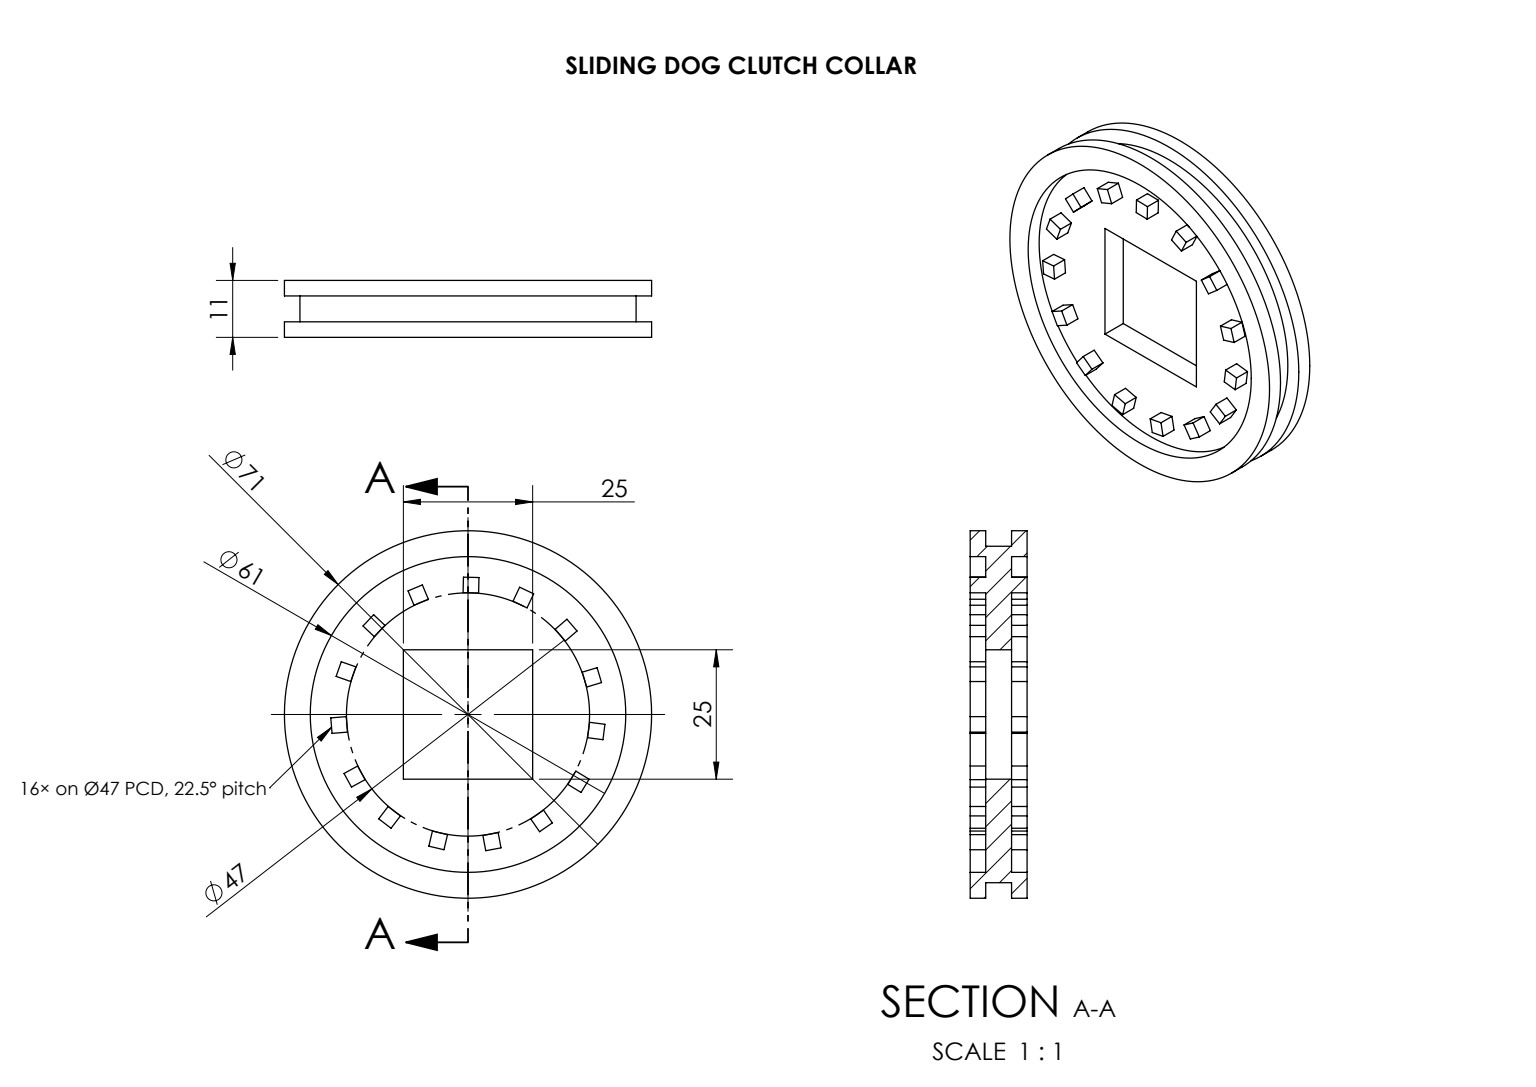
ISO-10303-21;
HEADER;
FILE_DESCRIPTION (('STEP AP214'),
    '1' );
FILE_NAME ('Sliding Dog Clutch Collar.step',
    '2026-10-08T09:53:37',
    ( '' ),
    ( '' ),
    'SwSTEP 2.0',
    'SolidWorks 2026',
    '' );
FILE_SCHEMA (( 'AUTOMOTIVE_DESIGN' ));
ENDSEC;

DATA;
#12=CARTESIAN_POINT ( 'NONE',  ( 20.85212586905262100, -130.9402397935870965, 2.500000000000000000 ) ) ;
#51=EDGE_CURVE ( 'NONE', #68933, #53084, #10085, .T. ) ;
#57=DIRECTION ( 'NONE',  ( -0.9966891607226785466, -0.08130631524009969413, 0.000000000000000000 ) ) ;
#59=DIRECTION ( 'NONE',  ( -0.3311129884571295534, -0.9435911131814398445, 0.000000000000000000 ) ) ;
#64=CARTESIAN_POINT ( 'NONE',  ( -26.29030328629083968, -123.6496510949466341, -5.500000000000000000 ) ) ;
#71=FACE_OUTER_BOUND ( 'NONE', #8361, .T. ) ;
#105=VERTEX_POINT ( 'NONE', #27751 ) ;
#152=CARTESIAN_POINT ( 'NONE',  ( -18.24502636017238899, -100.7225776329765665, 5.500000000000000000 ) ) ;
#170=ORIENTED_EDGE ( 'NONE', *, *, #48054, .T. ) ;
#195=DIRECTION ( 'NONE',  ( -0.000000000000000000, -0.000000000000000000, 1.000000000000000000 ) ) ;
#208=CARTESIAN_POINT ( 'NONE',  ( -0.7800914985199643992, -121.2811936832255100, 2.500000000000000000 ) ) ;
#210=CARTESIAN_POINT ( 'NONE',  ( 11.41210121379328335, -99.40233154247455616, 5.500000000000000000 ) ) ;
#218=EDGE_LOOP ( 'NONE', ( #22969, #71308, #32265, #23683 ) ) ;
#224=ADVANCED_FACE ( 'NONE', ( #20004 ), #64049, .F. ) ;
#245=VECTOR ( 'NONE', #9252, 1000.000000000000000 ) ;
#248=CARTESIAN_POINT ( 'NONE',  ( -16.06301359042743115, -102.7814171781257357, 2.500000000000000000 ) ) ;
#265=PLANE ( 'NONE',  #60728 ) ;
#266=CARTESIAN_POINT ( 'NONE',  ( -8.826826895187510402, -94.96827758698185562, 5.500000000000000000 ) ) ;
#268=ORIENTED_EDGE ( 'NONE', *, *, #56458, .T. ) ;
#303=EDGE_CURVE ( 'NONE', #64095, #48732, #3130, .T. ) ;
#384=CARTESIAN_POINT ( 'NONE',  ( 3.429551818649054340, -146.3199197248623875, 5.500000000000000000 ) ) ;
#386=LINE ( 'NONE', #68776, #73091 ) ;
#390=LINE ( 'NONE', #68413, #20038 ) ;
#395=CARTESIAN_POINT ( 'NONE',  ( 22.63442173698368620, -133.7816164738524378, -2.500000000000000000 ) ) ;
#401=ORIENTED_EDGE ( 'NONE', *, *, #30678, .T. ) ;
#481=FACE_OUTER_BOUND ( 'NONE', #34293, .T. ) ;
#549=DIRECTION ( 'NONE',  ( -0.3853207896976547642, 0.9227826878668540234, 0.000000000000000000 ) ) ;
#565=EDGE_CURVE ( 'NONE', #23559, #52552, #27876, .T. ) ;
#567=VECTOR ( 'NONE', #11381, 1000.000000000000000 ) ;
#580=FACE_OUTER_BOUND ( 'NONE', #12043, .T. ) ;
#591=CIRCLE ( 'NONE', #53356, 35.50000000000000711 ) ;
#648=FACE_OUTER_BOUND ( 'NONE', #4489, .T. ) ;
#656=EDGE_CURVE ( 'NONE', #45592, #59758, #43789, .T. ) ;
#726=CARTESIAN_POINT ( 'NONE',  ( 9.984461079971730157, -95.40710393340120277, 5.500000000000000000 ) ) ;
#739=CARTESIAN_POINT ( 'NONE',  ( -23.54415474984308787, -120.4156646670583086, 5.500000000000000000 ) ) ;
#753=CARTESIAN_POINT ( 'NONE',  ( 26.47460221209471598, -121.8961639463267090, 5.500000000000000000 ) ) ;
#776=EDGE_LOOP ( 'NONE', ( #60937, #39384, #65729, #18843 ) ) ;
#780=LINE ( 'NONE', #58251, #57390 ) ;
#809=CARTESIAN_POINT ( 'NONE',  ( -0.8815729230226008184, -93.47222532549339746, -5.500000000000000000 ) ) ;
#811=LINE ( 'NONE', #46635, #58781 ) ;
#837=PLANE ( 'NONE',  #5857 ) ;
#854=( NAMED_UNIT ( * ) SI_UNIT ( $, .STERADIAN. ) SOLID_ANGLE_UNIT ( ) );
#860=DIRECTION ( 'NONE',  ( -0.000000000000000000, -0.000000000000000000, -1.000000000000000000 ) ) ;
#883=EDGE_CURVE ( 'NONE', #14710, #67113, #37603, .T. ) ;
#885=ORIENTED_EDGE ( 'NONE', *, *, #19699, .F. ) ;
#897=VECTOR ( 'NONE', #23392, 1000.000000000000000 ) ;
#904=DIRECTION ( 'NONE',  ( -1.000000000000000000, 0.000000000000000000, 0.000000000000000000 ) ) ;
#920=FACE_OUTER_BOUND ( 'NONE', #19157, .T. ) ;
#923=LINE ( 'NONE', #34721, #21582 ) ;
#930=VECTOR ( 'NONE', #45166, 1000.000000000000000 ) ;
#947=AXIS2_PLACEMENT_3D ( 'NONE', #33555, #73025, #5390 ) ;
#949=PLANE ( 'NONE',  #67943 ) ;
#957=ORIENTED_EDGE ( 'NONE', *, *, #41163, .T. ) ;
#967=AXIS2_PLACEMENT_3D ( 'NONE', #58203, #18343, #42767 ) ;
#973=VERTEX_POINT ( 'NONE', #6001 ) ;
#982=CARTESIAN_POINT ( 'NONE',  ( -24.50849501662245800, -109.8101191361138831, -2.500000000000000444 ) ) ;
#1018=DIRECTION ( 'NONE',  ( -0.000000000000000000, -0.000000000000000000, 1.000000000000000000 ) ) ;
#1038=VERTEX_POINT ( 'NONE', #45100 ) ;
#1040=ORIENTED_EDGE ( 'NONE', *, *, #39297, .F. ) ;
#1043=DIRECTION ( 'NONE',  ( -0.000000000000000000, -0.000000000000000000, 1.000000000000000000 ) ) ;
#1059=ORIENTED_EDGE ( 'NONE', *, *, #39337, .F. ) ;
#1087=CARTESIAN_POINT ( 'NONE',  ( 22.08297821871651934, -111.8242998470044540, 5.500000000000000000 ) ) ;
#1092=LINE ( 'NONE', #24349, #38349 ) ;
#1109=DIRECTION ( 'NONE',  ( -0.000000000000000000, -0.000000000000000000, -1.000000000000000000 ) ) ;
#1160=FACE_OUTER_BOUND ( 'NONE', #45975, .T. ) ;
#1173=VERTEX_POINT ( 'NONE', #12346 ) ;
#1184=EDGE_LOOP ( 'NONE', ( #11101, #10539, #73075, #4642 ) ) ;
#1199=VECTOR ( 'NONE', #23641, 1000.000000000000000 ) ;
#1219=CARTESIAN_POINT ( 'NONE',  ( 13.83832728059186046, -142.6495187161941089, 5.500000000000000000 ) ) ;
#1231=ORIENTED_EDGE ( 'NONE', *, *, #64365, .F. ) ;
#1253=EDGE_CURVE ( 'NONE', #62521, #29721, #66451, .T. ) ;
#1266=EDGE_CURVE ( 'NONE', #63423, #62521, #21300, .T. ) ;
#1275=CARTESIAN_POINT ( 'NONE',  ( -16.07206065793331007, -141.0698568150738197, -2.500000000000000000 ) ) ;
#1279=ORIENTED_EDGE ( 'NONE', *, *, #2361, .T. ) ;
#1296=DIRECTION ( 'NONE',  ( -0.4279312458753000703, -0.9038112904824842087, 0.000000000000000000 ) ) ;
#1340=LINE ( 'NONE', #12563, #61150 ) ;
#1343=EDGE_LOOP ( 'NONE', ( #50298, #67195, #1354, #42780 ) ) ;
#1349=ORIENTED_EDGE ( 'NONE', *, *, #68241, .T. ) ;
#1354=ORIENTED_EDGE ( 'NONE', *, *, #44246, .T. ) ;
#1372=CARTESIAN_POINT ( 'NONE',  ( -7.572224309238338336, -145.4393675041377492, -2.500000000000000444 ) ) ;
#1380=VECTOR ( 'NONE', #34980, 1000.000000000000000 ) ;
#1381=ORIENTED_EDGE ( 'NONE', *, *, #5276, .T. ) ;
#1394=ADVANCED_FACE ( 'NONE', ( #38992 ), #12165, .F. ) ;
#1438=ORIENTED_EDGE ( 'NONE', *, *, #18270, .F. ) ;
#1485=LINE ( 'NONE', #36753, #73620 ) ;
#1487=LINE ( 'NONE', #13080, #23907 ) ;
#1521=AXIS2_PLACEMENT_3D ( 'NONE', #26148, #53617, #71638 ) ;
#1537=ORIENTED_EDGE ( 'NONE', *, *, #72023, .T. ) ;
#1539=EDGE_LOOP ( 'NONE', ( #2290, #72966 ) ) ;
#1553=CARTESIAN_POINT ( 'NONE',  ( -26.53422223201112828, -120.6595836127786043, 5.500000000000000000 ) ) ;
#1598=SURFACE_STYLE_USAGE ( .BOTH. , #12090 ) ;
#1599=ORIENTED_EDGE ( 'NONE', *, *, #38387, .F. ) ;
#1602=ORIENTED_EDGE ( 'NONE', *, *, #6612, .T. ) ;
#1625=ORIENTED_EDGE ( 'NONE', *, *, #25023, .F. ) ;
#1653=ORIENTED_EDGE ( 'NONE', *, *, #66798, .T. ) ;
#1676=AXIS2_PLACEMENT_3D ( 'NONE', #49631, #3078, #56026 ) ;
#1704=VERTEX_POINT ( 'NONE', #49333 ) ;
#1707=CARTESIAN_POINT ( 'NONE',  ( 0.4301293587033142574, -121.4370068666438556, -2.500000000000000000 ) ) ;
#1722=CARTESIAN_POINT ( 'NONE',  ( -22.53294031248081808, -134.0273518838794757, -2.500000000000000000 ) ) ;
#1723=ORIENTED_EDGE ( 'NONE', *, *, #48136, .T. ) ;
#1748=CARTESIAN_POINT ( 'NONE',  ( 10.05638427806949586, -98.76043467366159234, 2.500000000000000000 ) ) ;
#1754=CARTESIAN_POINT ( 'NONE',  ( 4.903647372192503795, -146.0423547792665886, -2.500000000000000000 ) ) ;
#1765=AXIS2_PLACEMENT_3D ( 'NONE', #44988, #68289, #73165 ) ;
#1781=VERTEX_POINT ( 'NONE', #33901 ) ;
#1784=VECTOR ( 'NONE', #5629, 1000.000000000000000 ) ;
#1785=CARTESIAN_POINT ( 'NONE',  ( 30.50000000000000000, -120.0000000000000000, 2.500000000000000000 ) ) ;
#1811=ORIENTED_EDGE ( 'NONE', *, *, #51766, .F. ) ;
#1826=ORIENTED_EDGE ( 'NONE', *, *, #3341, .T. ) ;
#1835=CARTESIAN_POINT ( 'NONE',  ( -26.53422223201112828, -120.6595836127786043, 5.500000000000000000 ) ) ;
#1837=ORIENTED_EDGE ( 'NONE', *, *, #48323, .F. ) ;
#1839=DIRECTION ( 'NONE',  ( -0.7585478161175706058, -0.6516173805718078471, 0.000000000000000000 ) ) ;
#1842=FACE_OUTER_BOUND ( 'NONE', #73904, .T. ) ;
#1847=DIRECTION ( 'NONE',  ( 0.5200609990132993854, 0.8541291221503275466, -0.000000000000000000 ) ) ;
#1885=EDGE_LOOP ( 'NONE', ( #9049, #54453, #6920, #47224 ) ) ;
#1908=FACE_BOUND ( 'NONE', #36354, .T. ) ;
#1909=DIRECTION ( 'NONE',  ( -0.6862798483830533369, -0.7273375899149812085, 0.000000000000000000 ) ) ;
#1931=CARTESIAN_POINT ( 'NONE',  ( -0.8815729230226008184, -93.47222532549339746, 5.500000000000000000 ) ) ;
#1939=CARTESIAN_POINT ( 'NONE',  ( -18.12185313557660038, -104.9634299478706794, 5.500000000000000000 ) ) ;
#1956=CARTESIAN_POINT ( 'NONE',  ( -22.67106064244953245, -113.6342314410295842, 2.500000000000000000 ) ) ;
#1959=EDGE_LOOP ( 'NONE', ( #56725, #22128, #74154, #73797 ) ) ;
#1966=VERTEX_POINT ( 'NONE', #2696 ) ;
#1969=ORIENTED_EDGE ( 'NONE', *, *, #5881, .F. ) ;
#1977=ADVANCED_FACE ( 'NONE', ( #41753 ), #7186, .T. ) ;
#2011=EDGE_CURVE ( 'NONE', #44097, #4558, #30834, .T. ) ;
#2015=DIRECTION ( 'NONE',  ( -0.7585478161175716050, -0.6516173805718067369, 0.000000000000000000 ) ) ;
#2029=CARTESIAN_POINT ( 'NONE',  ( -23.30023580412278505, -123.4057321492263384, 5.500000000000000000 ) ) ;
#2040=FILL_AREA_STYLE_COLOUR ( '', #49372 ) ;
#2043=CARTESIAN_POINT ( 'NONE',  ( -11.59517495878806947, -96.12423995607481686, 5.500000000000000000 ) ) ;
#2082=ORIENTED_EDGE ( 'NONE', *, *, #60638, .T. ) ;
#2084=CARTESIAN_POINT ( 'NONE',  ( 0.6180191030787338669, -93.50720753887522108, -2.500000000000000000 ) ) ;
#2101=CARTESIAN_POINT ( 'NONE',  ( -24.94940289813038703, -237.3777120880567963, 5.500000000000000000 ) ) ;
#2107=EDGE_CURVE ( 'NONE', #22856, #34880, #48875, .T. ) ;
#2113=EDGE_CURVE ( 'NONE', #8769, #59758, #72169, .T. ) ;
#2145=ORIENTED_EDGE ( 'NONE', *, *, #64889, .T. ) ;
#2160=CARTESIAN_POINT ( 'NONE',  ( -26.29030328629083968, -123.6496510949466341, 2.500000000000000000 ) ) ;
#2173=CARTESIAN_POINT ( 'NONE',  ( 23.41451323550360186, -132.5004227906269989, -5.500000000000000000 ) ) ;
#2175=CARTESIAN_POINT ( 'NONE',  ( -1.384174031800281979, -120.5779811845464735, -2.500000000000000000 ) ) ;
#2189=DIRECTION ( 'NONE',  ( -0.9918136447140100120, 0.1276937514489704939, 0.000000000000000000 ) ) ;
#2197=ORIENTED_EDGE ( 'NONE', *, *, #69129, .F. ) ;
#2202=ORIENTED_EDGE ( 'NONE', *, *, #62936, .T. ) ;
#2290=ORIENTED_EDGE ( 'NONE', *, *, #74029, .F. ) ;
#2315=CARTESIAN_POINT ( 'NONE',  ( -15.44521549751111955, -137.7748507232956001, -2.500000000000000000 ) ) ;
#2321=EDGE_CURVE ( 'NONE', #28941, #7487, #57491, .T. ) ;
#2322=ADVANCED_FACE ( 'NONE', ( #73654 ), #10891, .F. ) ;
#2326=PLANE ( 'NONE',  #26246 ) ;
#2329=CARTESIAN_POINT ( 'NONE',  ( -20.30386590532155111, -102.9045904027214959, -2.500000000000000000 ) ) ;
#2332=VECTOR ( 'NONE', #7775, 1000.000000000000114 ) ;
#2351=CARTESIAN_POINT ( 'NONE',  ( -20.30386590532152979, -102.9045904027214959, 5.500000000000000000 ) ) ;
#2360=VECTOR ( 'NONE', #38026, 1000.000000000000000 ) ;
#2361=EDGE_CURVE ( 'NONE', #54121, #6591, #390, .T. ) ;
#2369=FACE_OUTER_BOUND ( 'NONE', #40880, .T. ) ;
#2372=ORIENTED_EDGE ( 'NONE', *, *, #7575, .T. ) ;
#2386=DIRECTION ( 'NONE',  ( -0.000000000000000000, -0.000000000000000000, -1.000000000000000000 ) ) ;
#2405=DIRECTION ( 'NONE',  ( -0.6862798483830533369, -0.7273375899149812085, 0.000000000000000000 ) ) ;
#2427=CARTESIAN_POINT ( 'NONE',  ( 24.94940289813197509, -237.3777120880564553, -5.500000000000000000 ) ) ;
#2428=DIRECTION ( 'NONE',  ( 0.6064928550163524168, 0.7950889364178788110, -0.000000000000000000 ) ) ;
#2467=DIRECTION ( 'NONE',  ( -0.000000000000000000, -0.000000000000000000, -1.000000000000000000 ) ) ;
#2505=EDGE_CURVE ( 'NONE', #6335, #6594, #41666, .T. ) ;
#2541=CARTESIAN_POINT ( 'NONE',  ( -0.7800914985199643992, -121.2811936832255100, -2.500000000000000000 ) ) ;
#2561=LINE ( 'NONE', #48369, #245 ) ;
#2568=DIRECTION ( 'NONE',  ( 0.3090169943749448977, 0.9510565162951543083, 0.000000000000000000 ) ) ;
#2579=LINE ( 'NONE', #1835, #53727 ) ;
#2597=CARTESIAN_POINT ( 'NONE',  ( -23.54415474984308432, -120.4156646670583086, -2.500000000000000000 ) ) ;
#2615=ADVANCED_FACE ( 'NONE', ( #26957 ), #2964, .F. ) ;
#2624=DIRECTION ( 'NONE',  ( -0.2867529058022035837, 0.9580045777625452175, 0.000000000000000000 ) ) ;
#2634=ORIENTED_EDGE ( 'NONE', *, *, #24041, .F. ) ;
#2635=CARTESIAN_POINT ( 'NONE',  ( 12.13205353604972991, -140.1820037904669789, 5.500000000000000000 ) ) ;
#2639=CARTESIAN_POINT ( 'NONE',  ( -3.961125083139900749, -143.2122702051246677, 5.500000000000000000 ) ) ;
#2641=CARTESIAN_POINT ( 'NONE',  ( 12.13205353604972991, -140.1820037904669789, 5.500000000000000000 ) ) ;
#2654=VERTEX_POINT ( 'NONE', #43173 ) ;
#2667=DIRECTION ( 'NONE',  ( -0.1850432970638682395, 0.9827303690289280746, 0.000000000000000000 ) ) ;
#2671=EDGE_CURVE ( 'NONE', #22209, #16806, #61189, .T. ) ;
#2689=CARTESIAN_POINT ( 'NONE',  ( 32.50000000000000000, -120.0000000000000000, 2.500000000000000000 ) ) ;
#2696=CARTESIAN_POINT ( 'NONE',  ( 24.95699195200416654, -110.9640411295978595, 2.500000000000000000 ) ) ;
#2712=CARTESIAN_POINT ( 'NONE',  ( -0.1219594728601508804, -118.5049662589159567, -2.500000000000000000 ) ) ;
#2717=DIRECTION ( 'NONE',  ( -0.000000000000000000, -0.000000000000000000, -1.000000000000000000 ) ) ;
#2726=EDGE_LOOP ( 'NONE', ( #54837, #44802, #69623, #30782 ) ) ;
#2730=EDGE_LOOP ( 'NONE', ( #43648, #11853, #10232, #41324 ) ) ;
#2752=FACE_OUTER_BOUND ( 'NONE', #72336, .T. ) ;
#2755=DIRECTION ( 'NONE',  ( 0.02332147558787931590, 0.9997280174009348652, -0.000000000000000000 ) ) ;
#2758=EDGE_CURVE ( 'NONE', #7483, #63916, #28822, .T. ) ;
#2759=CARTESIAN_POINT ( 'NONE',  ( 0.9774260708577211521, -121.1378217241763622, 2.500000000000000000 ) ) ;
#2762=ORIENTED_EDGE ( 'NONE', *, *, #2758, .T. ) ;
#2775=DIRECTION ( 'NONE',  ( 0.000000000000000000, 0.000000000000000000, -1.000000000000000000 ) ) ;
#2784=CARTESIAN_POINT ( 'NONE',  ( 21.07894319797337701, -103.8699611390234878, -5.500000000000000000 ) ) ;
#2800=VERTEX_POINT ( 'NONE', #21694 ) ;
#2808=ORIENTED_EDGE ( 'NONE', *, *, #40826, .F. ) ;
#2845=ORIENTED_EDGE ( 'NONE', *, *, #10162, .F. ) ;
#2868=AXIS2_PLACEMENT_3D ( 'NONE', #12120, #35427, #47091 ) ;
#2902=VERTEX_POINT ( 'NONE', #45779 ) ;
#2915=DIRECTION ( 'NONE',  ( -0.000000000000000000, -0.000000000000000000, -1.000000000000000000 ) ) ;
#2924=CARTESIAN_POINT ( 'NONE',  ( -30.50000000000000000, -120.0000000000000000, 2.500000000000000000 ) ) ;
#2944=CARTESIAN_POINT ( 'NONE',  ( -20.62008904684763166, -131.2721749321093512, 2.500000000000000000 ) ) ;
#2957=EDGE_CURVE ( 'NONE', #62465, #52552, #27369, .T. ) ;
#2964=PLANE ( 'NONE',  #49843 ) ;
#2978=DIRECTION ( 'NONE',  ( 0.9580045777625452175, 0.2867529058022035837, -0.000000000000000000 ) ) ;
#2990=DIRECTION ( 'NONE',  ( -0.7950889364178798102, 0.6064928550163511956, 0.000000000000000000 ) ) ;
#3010=ORIENTED_EDGE ( 'NONE', *, *, #53161, .F. ) ;
#3022=VERTEX_POINT ( 'NONE', #62360 ) ;
#3034=CARTESIAN_POINT ( 'NONE',  ( 26.09152095774781799, -124.8716048804687375, 5.500000000000000000 ) ) ;
#3036=LINE ( 'NONE', #9373, #47208 ) ;
#3037=CARTESIAN_POINT ( 'NONE',  ( 13.83832728059186046, -142.6495187161941089, -5.500000000000000000 ) ) ;
#3045=FACE_OUTER_BOUND ( 'NONE', #46790, .T. ) ;
#3051=ORIENTED_EDGE ( 'NONE', *, *, #65354, .T. ) ;
#3078=DIRECTION ( 'NONE',  ( 0.7585478161175706058, 0.6516173805718080692, -0.000000000000000000 ) ) ;
#3096=ORIENTED_EDGE ( 'NONE', *, *, #22042, .T. ) ;
#3099=LINE ( 'NONE', #53462, #15602 ) ;
#3103=EDGE_CURVE ( 'NONE', #27761, #71554, #57819, .T. ) ;
#3126=CARTESIAN_POINT ( 'NONE',  ( 21.07894319797337701, -103.8699611390234878, 5.500000000000000000 ) ) ;
#3130=LINE ( 'NONE', #61360, #42832 ) ;
#3142=CARTESIAN_POINT ( 'NONE',  ( 21.07894319797337701, -103.8699611390234878, 5.500000000000000000 ) ) ;
#3144=LINE ( 'NONE', #43723, #13744 ) ;
#3149=ORIENTED_EDGE ( 'NONE', *, *, #18241, .F. ) ;
#3158=VERTEX_POINT ( 'NONE', #70180 ) ;
#3176=CARTESIAN_POINT ( 'NONE',  ( 18.80329974962065265, -105.8248132807389084, 5.500000000000000000 ) ) ;
#3180=CARTESIAN_POINT ( 'NONE',  ( 22.94323693612312809, -114.6983135802921083, 5.500000000000000000 ) ) ;
#3191=EDGE_CURVE ( 'NONE', #20908, #68902, #3286, .T. ) ;
#3210=EDGE_LOOP ( 'NONE', ( #28468, #25337, #66049, #46841 ) ) ;
#3218=ORIENTED_EDGE ( 'NONE', *, *, #2113, .F. ) ;
#3237=LINE ( 'NONE', #14855, #10050 ) ;
#3254=LINE ( 'NONE', #59262, #45303 ) ;
#3256=PLANE ( 'NONE',  #1521 ) ;
#3264=EDGE_LOOP ( 'NONE', ( #63569, #11796, #22892, #36153 ) ) ;
#3271=CARTESIAN_POINT ( 'NONE',  ( 12.13205353604972991, -140.1820037904669789, -5.500000000000000000 ) ) ;
#3284=EDGE_CURVE ( 'NONE', #38750, #8033, #66778, .T. ) ;
#3286=LINE ( 'NONE', #8149, #68208 ) ;
#3298=VECTOR ( 'NONE', #35506, 1000.000000000000000 ) ;
#3300=DIRECTION ( 'NONE',  ( -0.3311129884571295534, -0.9435911131814398445, 0.000000000000000000 ) ) ;
#3311=CARTESIAN_POINT ( 'NONE',  ( 0.7800914985199594032, -118.7188063167744900, 2.500000000000000000 ) ) ;
#3333=EDGE_CURVE ( 'NONE', #63423, #58064, #43504, .T. ) ;
#3339=VECTOR ( 'NONE', #3361, 1000.000000000000114 ) ;
#3341=EDGE_CURVE ( 'NONE', #51387, #24434, #32181, .T. ) ;
#3361=DIRECTION ( 'NONE',  ( 0.9227826878668540234, 0.3853207896976547087, -0.000000000000000000 ) ) ;
#3362=ORIENTED_EDGE ( 'NONE', *, *, #10881, .F. ) ;
#3386=CARTESIAN_POINT ( 'NONE',  ( 0.000000000000000000, 0.000000000000000000, -5.500000000000000000 ) ) ;
#3402=EDGE_CURVE ( 'NONE', #46548, #64355, #67522, .T. ) ;
#3431=FACE_BOUND ( 'NONE', #1885, .T. ) ;
#3445=VECTOR ( 'NONE', #58676, 1000.000000000000114 ) ;
#3468=CARTESIAN_POINT ( 'NONE',  ( -23.30023580412278861, -123.4057321492263384, -2.500000000000000000 ) ) ;
#3476=EDGE_LOOP ( 'NONE', ( #9812, #6944, #5386, #24783 ) ) ;
#3495=CARTESIAN_POINT ( 'NONE',  ( -12.50000000000000000, -107.5000000000000000, 2.500000000000000000 ) ) ;
#3507=PLANE ( 'NONE',  #24549 ) ;
#3519=DIRECTION ( 'NONE',  ( -0.000000000000000000, -0.000000000000000000, -1.000000000000000000 ) ) ;
#3526=EDGE_LOOP ( 'NONE', ( #43877, #10858, #22393, #6256 ) ) ;
#3529=EDGE_CURVE ( 'NONE', #65294, #46548, #73146, .T. ) ;
#3536=EDGE_LOOP ( 'NONE', ( #57725, #27089 ) ) ;
#3549=VECTOR ( 'NONE', #50670, 1000.000000000000000 ) ;
#3571=LINE ( 'NONE', #71209, #52794 ) ;
#3582=DIRECTION ( 'NONE',  ( -0.6516173805718079581, 0.7585478161175704948, 0.000000000000000000 ) ) ;
#3592=EDGE_CURVE ( 'NONE', #14025, #14710, #46080, .T. ) ;
#3598=LINE ( 'NONE', #66002, #53293 ) ;
#3615=EDGE_CURVE ( 'NONE', #14221, #69250, #35890, .T. ) ;
#3649=CARTESIAN_POINT ( 'NONE',  ( 1.029419772574596825, -118.9089936151275140, -2.500000000000000000 ) ) ;
#3677=DIRECTION ( 'NONE',  ( -0.000000000000000000, -0.000000000000000000, -1.000000000000000000 ) ) ;
#3684=CARTESIAN_POINT ( 'NONE',  ( -23.42219527698293646, -121.9106984081423803, -2.500000000000000000 ) ) ;
#3718=EDGE_LOOP ( 'NONE', ( #6494, #39883, #7441, #3218 ) ) ;
#3726=VERTEX_POINT ( 'NONE', #43778 ) ;
#3735=CIRCLE ( 'NONE', #48154, 32.50000000000000000 ) ;
#3745=EDGE_LOOP ( 'NONE', ( #41723, #41040, #62519, #34905 ) ) ;
#3778=CARTESIAN_POINT ( 'NONE',  ( 35.50000000000000711, -120.0000000000000000, 2.500000000000000000 ) ) ;
#3794=EDGE_LOOP ( 'NONE', ( #37080, #23623, #12025, #62762 ) ) ;
#3827=DIRECTION ( 'NONE',  ( 0.1850432970638656860, -0.9827303690289285187, 0.000000000000000000 ) ) ;
#3829=CARTESIAN_POINT ( 'NONE',  ( -18.24502636017238899, -100.7225776329765665, 5.500000000000000000 ) ) ;
#3836=CARTESIAN_POINT ( 'NONE',  ( 25.81725066941077529, -113.8380548628854854, 5.500000000000000000 ) ) ;
#3870=EDGE_CURVE ( 'NONE', #55006, #43075, #3735, .T. ) ;
#3887=CARTESIAN_POINT ( 'NONE',  ( -10.43921258969510824, -98.89258801967538659, 5.500000000000000000 ) ) ;
#3892=AXIS2_PLACEMENT_3D ( 'NONE', #61637, #9380, #39079 ) ;
#3908=EDGE_LOOP ( 'NONE', ( #42750, #9621 ) ) ;
#3938=CARTESIAN_POINT ( 'NONE',  ( -18.12185313557660038, -104.9634299478706794, 5.500000000000000000 ) ) ;
#3971=VECTOR ( 'NONE', #31374, 1000.000000000000000 ) ;
#3977=ORIENTED_EDGE ( 'NONE', *, *, #66110, .F. ) ;
#3981=EDGE_LOOP ( 'NONE', ( #42997, #28643, #28390, #44014 ) ) ;
#3994=EDGE_CURVE ( 'NONE', #63158, #20698, #12504, .T. ) ;
#4018=VECTOR ( 'NONE', #69227, 1000.000000000000000 ) ;
#4036=FACE_OUTER_BOUND ( 'NONE', #4823, .T. ) ;
#4042=EDGE_CURVE ( 'NONE', #23530, #42393, #39793, .T. ) ;
#4054=CARTESIAN_POINT ( 'NONE',  ( 0.5480546763151027401, -96.50639159107802811, -2.500000000000000000 ) ) ;
#4072=EDGE_CURVE ( 'NONE', #40306, #13957, #7249, .T. ) ;
#4090=DIRECTION ( 'NONE',  ( -0.2867529058022035837, 0.9580045777625452175, 0.000000000000000000 ) ) ;
#4157=VERTEX_POINT ( 'NONE', #3468 ) ;
#4169=EDGE_CURVE ( 'NONE', #35224, #26348, #9083, .T. ) ;
#4181=ORIENTED_EDGE ( 'NONE', *, *, #62951, .F. ) ;
#4188=VECTOR ( 'NONE', #2189, 1000.000000000000227 ) ;
#4218=DIRECTION ( 'NONE',  ( 0.9966891607226785466, 0.08130631524010119293, -0.000000000000000000 ) ) ;
#4245=DIRECTION ( 'NONE',  ( 1.000000000000000000, 0.000000000000000000, 0.000000000000000000 ) ) ;
#4258=ADVANCED_FACE ( 'NONE', ( #44047 ), #21846, .F. ) ;
#4260=DIRECTION ( 'NONE',  ( 0.9135454576426004225, 0.4067366430758009854, 0.000000000000000000 ) ) ;
#4266=CARTESIAN_POINT ( 'NONE',  ( 2.117611129180199558, -93.54218975225703048, 5.500000000000000000 ) ) ;
#4272=CARTESIAN_POINT ( 'NONE',  ( -35.50000000000000711, -120.0000000000000000, 5.500000000000000000 ) ) ;
#4282=VECTOR ( 'NONE', #73942, 1000.000000000000227 ) ;
#4316=FACE_OUTER_BOUND ( 'NONE', #44759, .T. ) ;
#4324=DIRECTION ( 'NONE',  ( -0.000000000000000000, -0.000000000000000000, -1.000000000000000000 ) ) ;
#4338=ADVANCED_FACE ( 'NONE', ( #9451 ), #61708, .F. ) ;
#4347=CARTESIAN_POINT ( 'NONE',  ( 5.822613034544236399, -142.8165987265839760, 5.500000000000000000 ) ) ;
#4427=DIRECTION ( 'NONE',  ( 0.9227826878668540234, 0.3853207896976547087, -0.000000000000000000 ) ) ;
#4455=CARTESIAN_POINT ( 'NONE',  ( 13.83832728059186046, -142.6495187161941089, 5.500000000000000000 ) ) ;
#4485=LINE ( 'NONE', #15363, #4789 ) ;
#4486=FACE_OUTER_BOUND ( 'NONE', #74137, .T. ) ;
#4489=EDGE_LOOP ( 'NONE', ( #46240, #12111, #67970, #67216 ) ) ;
#4513=EDGE_CURVE ( 'NONE', #67963, #12692, #37216, .T. ) ;
#4547=CARTESIAN_POINT ( 'NONE',  ( -6.880223345695647197, -142.5202692415819854, 5.500000000000000000 ) ) ;
#4554=ORIENTED_EDGE ( 'NONE', *, *, #68957, .T. ) ;
#4557=ORIENTED_EDGE ( 'NONE', *, *, #66619, .T. ) ;
#4558=VERTEX_POINT ( 'NONE', #47380 ) ;
#4567=CARTESIAN_POINT ( 'NONE',  ( 6.377742925735834234, -145.7647898336708181, 5.500000000000000000 ) ) ;
#4570=VECTOR ( 'NONE', #45189, 1000.000000000000114 ) ;
#4601=ADVANCED_FACE ( 'NONE', ( #48844 ), #66162, .F. ) ;
#4621=VECTOR ( 'NONE', #15272, 1000.000000000000114 ) ;
#4635=CARTESIAN_POINT ( 'NONE',  ( -48.80839716909612491, -10.37454508288793065, -5.500000000000000000 ) ) ;
#4637=CARTESIAN_POINT ( 'NONE',  ( -20.62008904684763166, -131.2721749321093512, -2.500000000000000000 ) ) ;
#4642=ORIENTED_EDGE ( 'NONE', *, *, #10287, .T. ) ;
#4661=CARTESIAN_POINT ( 'NONE',  ( 1.499592026101426168, -120.0349822133818094, -2.500000000000000000 ) ) ;
#4679=VECTOR ( 'NONE', #40232, 1000.000000000000000 ) ;
#4696=DIRECTION ( 'NONE',  ( 0.9997280174009349762, -0.02332147558787674158, 0.000000000000000000 ) ) ;
#4698=DIRECTION ( 'NONE',  ( 0.000000000000000000, 1.000000000000000000, 0.000000000000000000 ) ) ;
#4705=EDGE_CURVE ( 'NONE', #30043, #52797, #26653, .T. ) ;
#4714=DIRECTION ( 'NONE',  ( 0.000000000000000000, -0.000000000000000000, 1.000000000000000000 ) ) ;
#4722=CARTESIAN_POINT ( 'NONE',  ( -35.50000000000000711, -120.0000000000000000, -5.500000000000000000 ) ) ;
#4776=EDGE_CURVE ( 'NONE', #1966, #43631, #31922, .T. ) ;
#4789=VECTOR ( 'NONE', #48838, 1000.000000000000000 ) ;
#4793=LINE ( 'NONE', #21290, #39538 ) ;
#4797=CARTESIAN_POINT ( 'NONE',  ( 0.000000000000000000, -120.0000000000000000, 2.500000000000000000 ) ) ;
#4805=CARTESIAN_POINT ( 'NONE',  ( 12.50000000000000000, -107.5000000000000000, 2.500000000000000000 ) ) ;
#4816=LINE ( 'NONE', #32970, #33573 ) ;
#4823=EDGE_LOOP ( 'NONE', ( #70800, #29051, #11659, #42017 ) ) ;
#4861=DIRECTION ( 'NONE',  ( -0.02332147558787823691, -0.9997280174009349762, 0.000000000000000000 ) ) ;
#4874=EDGE_LOOP ( 'NONE', ( #43949, #50686, #42365, #54032 ) ) ;
#4879=VECTOR ( 'NONE', #35632, 1000.000000000000000 ) ;
#4911=DIRECTION ( 'NONE',  ( 0.9827303690289282967, 0.1850432970638667407, -0.000000000000000000 ) ) ;
#4941=VECTOR ( 'NONE', #37203, 1000.000000000000114 ) ;
#4945=FACE_OUTER_BOUND ( 'NONE', #3536, .T. ) ;
#4964=CARTESIAN_POINT ( 'NONE',  ( -1.355716935723729089, -119.3581031311870362, -2.500000000000000000 ) ) ;
#5004=FACE_OUTER_BOUND ( 'NONE', #41187, .T. ) ;
#5005=ORIENTED_EDGE ( 'NONE', *, *, #25811, .F. ) ;
#5006=LINE ( 'NONE', #4637, #7197 ) ;
#5008=ORIENTED_EDGE ( 'NONE', *, *, #8201, .F. ) ;
#5041=ADVANCED_FACE ( 'NONE', ( #20089 ), #9561, .T. ) ;
#5044=DIRECTION ( 'NONE',  ( 0.000000000000000000, 0.000000000000000000, 1.000000000000000000 ) ) ;
#5045=DIRECTION ( 'NONE',  ( 0.02332147558787822997, 0.9997280174009349762, 0.000000000000000000 ) ) ;
#5048=CARTESIAN_POINT ( 'NONE',  ( -13.05994868825747446, -139.5943292883446532, -5.500000000000000000 ) ) ;
#5067=DIRECTION ( 'NONE',  ( 0.7585478161175723821, 0.6516173805718057377, 0.000000000000000000 ) ) ;
#5082=FACE_OUTER_BOUND ( 'NONE', #19163, .T. ) ;
#5083=CARTESIAN_POINT ( 'NONE',  ( 19.12409105625795291, -101.5943176906707919, 2.500000000000000000 ) ) ;
#5098=EDGE_LOOP ( 'NONE', ( #27168, #7224, #66127, #58066 ) ) ;
#5102=EDGE_CURVE ( 'NONE', #40486, #17454, #32480, .T. ) ;
#5116=CARTESIAN_POINT ( 'NONE',  ( 2.117611129180199558, -93.54218975225703048, 2.500000000000000000 ) ) ;
#5137=DIRECTION ( 'NONE',  ( 0.08130631524010120681, -0.9966891607226784355, 0.000000000000000000 ) ) ;
#5162=FACE_OUTER_BOUND ( 'NONE', #11175, .T. ) ;
#5198=DIRECTION ( 'NONE',  ( -1.000000000000000000, 0.000000000000000000, 0.000000000000000000 ) ) ;
#5201=ORIENTED_EDGE ( 'NONE', *, *, #21799, .T. ) ;
#5210=ORIENTED_EDGE ( 'NONE', *, *, #56209, .F. ) ;
#5232=ORIENTED_EDGE ( 'NONE', *, *, #67900, .T. ) ;
#5264=VECTOR ( 'NONE', #57386, 1000.000000000000000 ) ;
#5268=ORIENTED_EDGE ( 'NONE', *, *, #30286, .T. ) ;
#5274=EDGE_CURVE ( 'NONE', #69665, #1704, #28322, .T. ) ;
#5276=EDGE_CURVE ( 'NONE', #43742, #6773, #39994, .T. ) ;
#5281=CARTESIAN_POINT ( 'NONE',  ( -3.961125083139900749, -143.2122702051246677, 5.500000000000000000 ) ) ;
#5284=PLANE ( 'NONE',  #58151 ) ;
#5299=EDGE_CURVE ( 'NONE', #49118, #68933, #12879, .T. ) ;
#5301=DIRECTION ( 'NONE',  ( 0.9227826878668540234, 0.3853207896976547087, 0.000000000000000000 ) ) ;
#5320=ORIENTED_EDGE ( 'NONE', *, *, #3333, .F. ) ;
#5355=CARTESIAN_POINT ( 'NONE',  ( -0.9515373497862389396, -96.47140937769621871, 5.500000000000000000 ) ) ;
#5366=LINE ( 'NONE', #57223, #36039 ) ;
#5374=VECTOR ( 'NONE', #24707, 1000.000000000000000 ) ;
#5386=ORIENTED_EDGE ( 'NONE', *, *, #59816, .T. ) ;
#5390=DIRECTION ( 'NONE',  ( 0.3090169943749448977, 0.9510565162951543083, 0.000000000000000000 ) ) ;
#5424=ORIENTED_EDGE ( 'NONE', *, *, #21799, .F. ) ;
#5429=LINE ( 'NONE', #56556, #54340 ) ;
#5451=ORIENTED_EDGE ( 'NONE', *, *, #23662, .T. ) ;
#5455=AXIS2_PLACEMENT_3D ( 'NONE', #15260, #20537, #66043 ) ;
#5482=ORIENTED_EDGE ( 'NONE', *, *, #59825, .T. ) ;
#5509=DIRECTION ( 'NONE',  ( -0.08130631524010122069, 0.9966891607226784355, 0.000000000000000000 ) ) ;
#5522=VECTOR ( 'NONE', #2467, 1000.000000000000000 ) ;
#5582=CARTESIAN_POINT ( 'NONE',  ( -6.880223345695647197, -142.5202692415819854, 5.500000000000000000 ) ) ;
#5598=MECHANICAL_DESIGN_GEOMETRIC_PRESENTATION_REPRESENTATION('',(#65580),#70381);
#5629=DIRECTION ( 'NONE',  ( -0.5200609990132993854, -0.8541291221503274356, 0.000000000000000000 ) ) ;
#5642=DIRECTION ( 'NONE',  ( 0.8225049752423776450, 0.5687579148473765889, 0.000000000000000000 ) ) ;
#5644=EDGE_CURVE ( 'NONE', #24488, #40794, #9465, .T. ) ;
#5651=LINE ( 'NONE', #5281, #46409 ) ;
#5653=CARTESIAN_POINT ( 'NONE',  ( 11.34017801569539685, -96.04900080221412395, -2.500000000000000000 ) ) ;
#5669=ORIENTED_EDGE ( 'NONE', *, *, #22611, .T. ) ;
#5697=ADVANCED_FACE ( 'NONE', ( #9840 ), #50431, .F. ) ;
#5721=FACE_OUTER_BOUND ( 'NONE', #29762, .T. ) ;
#5736=EDGE_LOOP ( 'NONE', ( #72619, #72189, #1969, #38688 ) ) ;
#5778=LINE ( 'NONE', #40346, #48742 ) ;
#5800=EDGE_CURVE ( 'NONE', #54047, #56693, #34250, .T. ) ;
#5805=VECTOR ( 'NONE', #17560, 1000.000000000000000 ) ;
#5846=ORIENTED_EDGE ( 'NONE', *, *, #42374, .F. ) ;
#5857=AXIS2_PLACEMENT_3D ( 'NONE', #46657, #29713, #16426 ) ;
#5874=ORIENTED_EDGE ( 'NONE', *, *, #62309, .T. ) ;
#5876=DIRECTION ( 'NONE',  ( 0.9918136447140100120, -0.1276937514489704939, 0.000000000000000000 ) ) ;
#5881=EDGE_CURVE ( 'NONE', #2902, #43742, #53033, .T. ) ;
#5892=DIRECTION ( 'NONE',  ( -0.9730327541852497042, 0.2306669878475623159, 0.000000000000000000 ) ) ;
#5907=FACE_OUTER_BOUND ( 'NONE', #21100, .T. ) ;
#5910=ORIENTED_EDGE ( 'NONE', *, *, #73650, .F. ) ;
#5939=AXIS2_PLACEMENT_3D ( 'NONE', #8152, #26555, #65679 ) ;
#5967=ORIENTED_EDGE ( 'NONE', *, *, #54804, .F. ) ;
#6001=CARTESIAN_POINT ( 'NONE',  ( 12.13205353604972991, -140.1820037904669789, -5.500000000000000000 ) ) ;
#6014=VECTOR ( 'NONE', #65712, 1000.000000000000114 ) ;
#6050=DIRECTION ( 'NONE',  ( 0.6862798483830533369, 0.7273375899149812085, 0.000000000000000000 ) ) ;
#6099=VECTOR ( 'NONE', #34440, 1000.000000000000114 ) ;
#6111=AXIS2_PLACEMENT_3D ( 'NONE', #23711, #51910, #68097 ) ;
#6122=AXIS2_PLACEMENT_3D ( 'NONE', #64241, #35642, #25115 ) ;
#6139=DIRECTION ( 'NONE',  ( -0.000000000000000000, -0.000000000000000000, 1.000000000000000000 ) ) ;
#6148=VERTEX_POINT ( 'NONE', #61267 ) ;
#6152=LINE ( 'NONE', #53108, #25932 ) ;
#6180=CARTESIAN_POINT ( 'NONE',  ( 0.000000000000000000, -120.0000000000000000, -5.500000000000000000 ) ) ;
#6205=VERTEX_POINT ( 'NONE', #67274 ) ;
#6217=ORIENTED_EDGE ( 'NONE', *, *, #15773, .T. ) ;
#6221=VECTOR ( 'NONE', #44219, 1000.000000000000000 ) ;
#6231=VERTEX_POINT ( 'NONE', #39825 ) ;
#6242=CARTESIAN_POINT ( 'NONE',  ( 22.08297821871651934, -111.8242998470044540, 5.500000000000000000 ) ) ;
#6244=EDGE_LOOP ( 'NONE', ( #72557, #32737, #74039, #58146 ) ) ;
#6249=DIRECTION ( 'NONE',  ( 0.6862798483830534479, 0.7273375899149810975, 0.000000000000000000 ) ) ;
#6252=CARTESIAN_POINT ( 'NONE',  ( 23.11608002360578240, -124.4885236261218182, 5.500000000000000000 ) ) ;
#6256=ORIENTED_EDGE ( 'NONE', *, *, #27249, .T. ) ;
#6266=DIRECTION ( 'NONE',  ( -0.8541291221503266584, 0.5200609990133008287, 0.000000000000000000 ) ) ;
#6278=VECTOR ( 'NONE', #30979, 1000.000000000000114 ) ;
#6287=DIRECTION ( 'NONE',  ( 0.3853207896976533209, -0.9227826878668545785, 0.000000000000000000 ) ) ;
#6294=FACE_OUTER_BOUND ( 'NONE', #28535, .T. ) ;
#6302=ORIENTED_EDGE ( 'NONE', *, *, #47419, .T. ) ;
#6305=VECTOR ( 'NONE', #12708, 999.9999999999998863 ) ;
#6329=CARTESIAN_POINT ( 'NONE',  ( -35.50000000000000711, -120.0000000000000000, 2.500000000000000000 ) ) ;
#6335=VERTEX_POINT ( 'NONE', #18349 ) ;
#6341=EDGE_LOOP ( 'NONE', ( #43867, #69874, #61233, #65500 ) ) ;
#6346=ORIENTED_EDGE ( 'NONE', *, *, #58664, .T. ) ;
#6347=ORIENTED_EDGE ( 'NONE', *, *, #50689, .F. ) ;
#6359=DIRECTION ( 'NONE',  ( 0.9827303690289279636, 0.1850432970638681840, 0.000000000000000000 ) ) ;
#6375=VECTOR ( 'NONE', #54688, 1000.000000000000114 ) ;
#6385=EDGE_CURVE ( 'NONE', #20073, #45219, #36014, .T. ) ;
#6386=ORIENTED_EDGE ( 'NONE', *, *, #11894, .T. ) ;
#6407=ORIENTED_EDGE ( 'NONE', *, *, #3333, .T. ) ;
#6411=CARTESIAN_POINT ( 'NONE',  ( 19.29194287201271862, -133.5026271600380880, 5.500000000000000000 ) ) ;
#6435=VECTOR ( 'NONE', #10581, 1000.000000000000000 ) ;
#6441=LINE ( 'NONE', #52287, #51855 ) ;
#6480=ORIENTED_EDGE ( 'NONE', *, *, #51624, .F. ) ;
#6494=ORIENTED_EDGE ( 'NONE', *, *, #68058, .T. ) ;
#6519=ORIENTED_EDGE ( 'NONE', *, *, #65201, .T. ) ;
#6525=EDGE_CURVE ( 'NONE', #22209, #69025, #1485, .T. ) ;
#6533=CARTESIAN_POINT ( 'NONE',  ( 0.000000000000000000, -120.0000000000000000, 2.500000000000000000 ) ) ;
#6554=VECTOR ( 'NONE', #47935, 1000.000000000000114 ) ;
#6560=ORIENTED_EDGE ( 'NONE', *, *, #60756, .T. ) ;
#6591=VERTEX_POINT ( 'NONE', #8927 ) ;
#6594=VERTEX_POINT ( 'NONE', #50624 ) ;
#6600=PLANE ( 'NONE',  #55460 ) ;
#6611=ORIENTED_EDGE ( 'NONE', *, *, #67291, .T. ) ;
#6612=EDGE_CURVE ( 'NONE', #29293, #4157, #26581, .T. ) ;
#6680=LINE ( 'NONE', #12678, #4188 ) ;
#6692=VECTOR ( 'NONE', #61445, 1000.000000000000114 ) ;
#6773=VERTEX_POINT ( 'NONE', #18266 ) ;
#6833=ORIENTED_EDGE ( 'NONE', *, *, #53751, .T. ) ;
#6871=DIRECTION ( 'NONE',  ( -0.000000000000000000, -0.000000000000000000, -1.000000000000000000 ) ) ;
#6892=DIRECTION ( 'NONE',  ( 1.000000000000000000, 0.000000000000000000, 0.000000000000000000 ) ) ;
#6900=DIRECTION ( 'NONE',  ( 0.9227826878668550226, 0.3853207896976523772, -0.000000000000000000 ) ) ;
#6920=ORIENTED_EDGE ( 'NONE', *, *, #40087, .T. ) ;
#6944=ORIENTED_EDGE ( 'NONE', *, *, #69129, .T. ) ;
#6967=EDGE_CURVE ( 'NONE', #40320, #37554, #13363, .T. ) ;
#6973=ORIENTED_EDGE ( 'NONE', *, *, #51766, .T. ) ;
#6980=FACE_OUTER_BOUND ( 'NONE', #1959, .T. ) ;
#6987=VECTOR ( 'NONE', #72351, 1000.000000000000227 ) ;
#6989=FACE_OUTER_BOUND ( 'NONE', #5098, .T. ) ;
#6995=VECTOR ( 'NONE', #21302, 1000.000000000000114 ) ;
#7009=CARTESIAN_POINT ( 'NONE',  ( 20.85212586905262100, -130.9402397935870965, 5.500000000000000000 ) ) ;
#7018=ORIENTED_EDGE ( 'NONE', *, *, #69502, .F. ) ;
#7020=ORIENTED_EDGE ( 'NONE', *, *, #3994, .T. ) ;
#7047=DIRECTION ( 'NONE',  ( -0.000000000000000000, -0.000000000000000000, -1.000000000000000000 ) ) ;
#7049=VECTOR ( 'NONE', #32393, 1000.000000000000000 ) ;
#7065=CARTESIAN_POINT ( 'NONE',  ( 21.07894319797337701, -103.8699611390234878, 5.500000000000000000 ) ) ;
#7067=EDGE_CURVE ( 'NONE', #4558, #6335, #3598, .T. ) ;
#7090=AXIS2_PLACEMENT_3D ( 'NONE', #36538, #70746, #20366 ) ;
#7100=ORIENTED_EDGE ( 'NONE', *, *, #14155, .F. ) ;
#7175=DIRECTION ( 'NONE',  ( -0.000000000000000000, -0.000000000000000000, 1.000000000000000000 ) ) ;
#7186=PLANE ( 'NONE',  #48860 ) ;
#7191=DIRECTION ( 'NONE',  ( 0.6691306063588671194, -0.7431448254773862505, 0.000000000000000000 ) ) ;
#7195=CARTESIAN_POINT ( 'NONE',  ( 114.1267819554180392, -82.91796067500511924, -5.500000000000000000 ) ) ;
#7196=EDGE_LOOP ( 'NONE', ( #71586, #7875, #7693, #18483 ) ) ;
#7197=VECTOR ( 'NONE', #16634, 1000.000000000000114 ) ;
#7221=ADVANCED_FACE ( 'NONE', ( #2369 ), #13230, .F. ) ;
#7224=ORIENTED_EDGE ( 'NONE', *, *, #15730, .T. ) ;
#7229=CARTESIAN_POINT ( 'NONE',  ( -22.67106064244953245, -113.6342314410295842, 5.500000000000000000 ) ) ;
#7243=ADVANCED_FACE ( 'NONE', ( #13952 ), #59846, .F. ) ;
#7249=LINE ( 'NONE', #63290, #13371 ) ;
#7258=ADVANCED_FACE ( 'NONE', ( #14340 ), #43308, .F. ) ;
#7261=LINE ( 'NONE', #70763, #68691 ) ;
#7313=ORIENTED_EDGE ( 'NONE', *, *, #56458, .F. ) ;
#7330=CARTESIAN_POINT ( 'NONE',  ( 4.348517481000897078, -143.0941636721797465, -2.500000000000000000 ) ) ;
#7339=DIRECTION ( 'NONE',  ( 0.9997280174009348652, -0.02332147558787931590, 0.000000000000000000 ) ) ;
#7346=VECTOR ( 'NONE', #67906, 1000.000000000000114 ) ;
#7370=DIRECTION ( 'NONE',  ( -0.8541291221503266584, 0.5200609990133008287, 0.000000000000000000 ) ) ;
#7372=( GEOMETRIC_REPRESENTATION_CONTEXT ( 3 ) GLOBAL_UNCERTAINTY_ASSIGNED_CONTEXT ( ( #66335 ) ) GLOBAL_UNIT_ASSIGNED_CONTEXT ( ( #47497, #41124, #23821 ) ) REPRESENTATION_CONTEXT ( 'NONE', 'WORKASPACE' ) );
#7382=VECTOR ( 'NONE', #70925, 1000.000000000000000 ) ;
#7387=VECTOR ( 'NONE', #2015, 1000.000000000000000 ) ;
#7416=ADVANCED_FACE ( 'NONE', ( #35264 ), #18700, .F. ) ;
#7425=DIRECTION ( 'NONE',  ( -0.000000000000000000, -0.000000000000000000, -1.000000000000000000 ) ) ;
#7435=AXIS2_PLACEMENT_3D ( 'NONE', #8067, #14816, #37763 ) ;
#7441=ORIENTED_EDGE ( 'NONE', *, *, #42983, .F. ) ;
#7443=AXIS2_PLACEMENT_3D ( 'NONE', #38948, #51326, #50964 ) ;
#7483=VERTEX_POINT ( 'NONE', #23993 ) ;
#7487=VERTEX_POINT ( 'NONE', #65326 ) ;
#7494=ORIENTED_EDGE ( 'NONE', *, *, #12997, .T. ) ;
#7502=VERTEX_POINT ( 'NONE', #47290 ) ;
#7511=FACE_BOUND ( 'NONE', #59973, .T. ) ;
#7530=DIRECTION ( 'NONE',  ( -0.4279312458752990711, -0.9038112904824846527, 0.000000000000000000 ) ) ;
#7546=PLANE ( 'NONE',  #36504 ) ;
#7561=CARTESIAN_POINT ( 'NONE',  ( -24.50849501662245800, -109.8101191361138831, 5.500000000000000000 ) ) ;
#7575=EDGE_CURVE ( 'NONE', #6594, #7502, #20564, .T. ) ;
#7590=ORIENTED_EDGE ( 'NONE', *, *, #38810, .T. ) ;
#7603=CARTESIAN_POINT ( 'NONE',  ( 89.17737905728634473, -39.70432723693593857, 5.500000000000000000 ) ) ;
#7627=DIRECTION ( 'NONE',  ( -0.000000000000000000, -0.000000000000000000, -1.000000000000000000 ) ) ;
#7631=ADVANCED_FACE ( 'NONE', ( #4036 ), #37120, .F. ) ;
#7649=CARTESIAN_POINT ( 'NONE',  ( -21.67772167707813935, -110.8034581014852762, 5.500000000000000000 ) ) ;
#7659=ORIENTED_EDGE ( 'NONE', *, *, #45769, .T. ) ;
#7664=EDGE_CURVE ( 'NONE', #1704, #54121, #8547, .T. ) ;
#7666=EDGE_LOOP ( 'NONE', ( #5210, #34211, #33527, #21898 ) ) ;
#7671=EDGE_LOOP ( 'NONE', ( #23753, #58367, #22947, #15159 ) ) ;
#7680=VERTEX_POINT ( 'NONE', #57011 ) ;
#7693=ORIENTED_EDGE ( 'NONE', *, *, #20646, .T. ) ;
#7707=VERTEX_POINT ( 'NONE', #73535 ) ;
#7710=ADVANCED_FACE ( 'NONE', ( #50229 ), #34066, .F. ) ;
#7724=ADVANCED_FACE ( 'NONE', ( #40446 ), #28419, .F. ) ;
#7773=FACE_OUTER_BOUND ( 'NONE', #9270, .T. ) ;
#7775=DIRECTION ( 'NONE',  ( -0.3853207896976523772, 0.9227826878668550226, 0.000000000000000000 ) ) ;
#7817=DIRECTION ( 'NONE',  ( -0.000000000000000000, -0.000000000000000000, -1.000000000000000000 ) ) ;
#7821=VECTOR ( 'NONE', #35894, 1000.000000000000114 ) ;
#7826=AXIS2_PLACEMENT_3D ( 'NONE', #6533, #27966, #57674 ) ;
#7844=ORIENTED_EDGE ( 'NONE', *, *, #17000, .T. ) ;
#7851=ORIENTED_EDGE ( 'NONE', *, *, #4072, .F. ) ;
#7860=CARTESIAN_POINT ( 'NONE',  ( -25.50183398199384754, -112.6408924756582053, 2.500000000000000000 ) ) ;
#7869=EDGE_CURVE ( 'NONE', #44533, #54089, #47568, .T. ) ;
#7871=FACE_BOUND ( 'NONE', #10810, .T. ) ;
#7874=VECTOR ( 'NONE', #37720, 1000.000000000000227 ) ;
#7875=ORIENTED_EDGE ( 'NONE', *, *, #55617, .T. ) ;
#7884=ORIENTED_EDGE ( 'NONE', *, *, #2505, .F. ) ;
#7892=EDGE_CURVE ( 'NONE', #53084, #44533, #59219, .T. ) ;
#7893=DIRECTION ( 'NONE',  ( -0.08130631524010117905, 0.9966891607226784355, 0.000000000000000000 ) ) ;
#7912=VECTOR ( 'NONE', #56680, 1000.000000000000000 ) ;
#7935=DIRECTION ( 'NONE',  ( 0.9966891607226785466, 0.08130631524009969413, -0.000000000000000000 ) ) ;
#8002=PLANE ( 'NONE',  #22666 ) ;
#8018=LINE ( 'NONE', #7649, #32962 ) ;
#8033=VERTEX_POINT ( 'NONE', #55052 ) ;
#8039=ORIENTED_EDGE ( 'NONE', *, *, #9754, .F. ) ;
#8043=ORIENTED_EDGE ( 'NONE', *, *, #8147, .T. ) ;
#8049=LINE ( 'NONE', #53925, #5522 ) ;
#8065=LINE ( 'NONE', #70840, #47513 ) ;
#8067=CARTESIAN_POINT ( 'NONE',  ( -18.12185313557660038, -104.9634299478706794, 5.500000000000000000 ) ) ;
#8069=LINE ( 'NONE', #70102, #7821 ) ;
#8075=AXIS2_PLACEMENT_3D ( 'NONE', #6180, #70394, #29438 ) ;
#8082=DIRECTION ( 'NONE',  ( -0.000000000000000000, -0.000000000000000000, 1.000000000000000000 ) ) ;
#8128=ORIENTED_EDGE ( 'NONE', *, *, #54812, .T. ) ;
#8147=EDGE_CURVE ( 'NONE', #12223, #6773, #38134, .T. ) ;
#8149=CARTESIAN_POINT ( 'NONE',  ( -1.459549131277904976, -119.6539995182286304, -2.500000000000000000 ) ) ;
#8152=CARTESIAN_POINT ( 'NONE',  ( 22.94323693612312809, -114.6983135802921083, 5.500000000000000000 ) ) ;
#8157=VERTEX_POINT ( 'NONE', #20841 ) ;
#8158=LINE ( 'NONE', #31087, #54189 ) ;
#8184=ORIENTED_EDGE ( 'NONE', *, *, #25650, .F. ) ;
#8191=ORIENTED_EDGE ( 'NONE', *, *, #33334, .T. ) ;
#8194=LINE ( 'NONE', #24026, #21549 ) ;
#8201=EDGE_CURVE ( 'NONE', #46993, #40794, #62187, .T. ) ;
#8208=PLANE ( 'NONE',  #47744 ) ;
#8236=PLANE ( 'NONE',  #73264 ) ;
#8238=FACE_BOUND ( 'NONE', #3264, .T. ) ;
#8240=ORIENTED_EDGE ( 'NONE', *, *, #9193, .T. ) ;
#8265=CARTESIAN_POINT ( 'NONE',  ( -11.59517495878806947, -96.12423995607481686, 5.500000000000000000 ) ) ;
#8271=CARTESIAN_POINT ( 'NONE',  ( -1.499592026101402853, -119.9650177866181764, 2.500000000000000000 ) ) ;
#8274=VECTOR ( 'NONE', #74247, 1000.000000000000114 ) ;
#8278=DIRECTION ( 'NONE',  ( 0.7950889364178788110, -0.6064928550163524168, 0.000000000000000000 ) ) ;
#8279=DIRECTION ( 'NONE',  ( -0.5200609990133016058, -0.8541291221503261033, 0.000000000000000000 ) ) ;
#8289=DIRECTION ( 'NONE',  ( 0.5687579148473765889, -0.8225049752423776450, 0.000000000000000000 ) ) ;
#8311=FACE_BOUND ( 'NONE', #11345, .T. ) ;
#8333=CARTESIAN_POINT ( 'NONE',  ( -7.670864526094549163, -97.73662565058241114, 5.500000000000000000 ) ) ;
#8350=PLANE ( 'NONE',  #7090 ) ;
#8356=AXIS2_PLACEMENT_3D ( 'NONE', #46183, #45828, #57837 ) ;
#8361=EDGE_LOOP ( 'NONE', ( #56133, #2202, #35775, #25883 ) ) ;
#8377=CARTESIAN_POINT ( 'NONE',  ( 0.000000000000000000, -89.50000000000000000, 5.500000000000000000 ) ) ;
#8390=ORIENTED_EDGE ( 'NONE', *, *, #30286, .F. ) ;
#8411=VECTOR ( 'NONE', #6249, 1000.000000000000114 ) ;
#8454=LINE ( 'NONE', #13704, #45777 ) ;
#8463=CARTESIAN_POINT ( 'NONE',  ( 16.84844760790522855, -103.5491698323862124, 5.500000000000000000 ) ) ;
#8467=PLANE ( 'NONE',  #73965 ) ;
#8477=DIRECTION ( 'NONE',  ( -0.5687579148473752566, 0.8225049752423786442, 0.000000000000000000 ) ) ;
#8481=DIRECTION ( 'NONE',  ( 0.6862798483830554463, 0.7273375899149793211, -0.000000000000000000 ) ) ;
#8491=ORIENTED_EDGE ( 'NONE', *, *, #44074, .F. ) ;
#8516=ADVANCED_FACE ( 'NONE', ( #32294 ), #47844, .F. ) ;
#8530=DIRECTION ( 'NONE',  ( -0.000000000000000000, -0.000000000000000000, -1.000000000000000000 ) ) ;
#8547=LINE ( 'NONE', #67914, #56952 ) ;
#8554=DIRECTION ( 'NONE',  ( 1.000000000000000000, 0.000000000000000000, 0.000000000000000000 ) ) ;
#8576=EDGE_CURVE ( 'NONE', #63916, #54914, #49226, .T. ) ;
#8587=ADVANCED_FACE ( 'NONE', ( #39073 ), #55614, .F. ) ;
#8606=DIRECTION ( 'NONE',  ( 0.6064928550163511956, 0.7950889364178798102, -0.000000000000000000 ) ) ;
#8609=ORIENTED_EDGE ( 'NONE', *, *, #29332, .T. ) ;
#8630=CARTESIAN_POINT ( 'NONE',  ( -23.25244084006223133, -132.7111759872722416, -2.500000000000000000 ) ) ;
#8647=DIRECTION ( 'NONE',  ( 0.9227826878668550226, 0.3853207896976523772, -0.000000000000000000 ) ) ;
#8678=ADVANCED_FACE ( 'NONE', ( #62390 ), #34169, .F. ) ;
#8686=DIRECTION ( 'NONE',  ( 0.000000000000000000, 0.000000000000000000, 1.000000000000000000 ) ) ;
#8703=DIRECTION ( 'NONE',  ( -0.9435911131814402886, 0.3311129884571281101, 0.000000000000000000 ) ) ;
#8717=VERTEX_POINT ( 'NONE', #12 ) ;
#8719=VECTOR ( 'NONE', #15278, 1000.000000000000000 ) ;
#8741=CARTESIAN_POINT ( 'NONE',  ( -24.50849501662245800, -109.8101191361138831, 5.500000000000000000 ) ) ;
#8747=DIRECTION ( 'NONE',  ( -0.000000000000000000, -0.000000000000000000, -1.000000000000000000 ) ) ;
#8748=FACE_OUTER_BOUND ( 'NONE', #19232, .T. ) ;
#8768=PLANE ( 'NONE',  #54724 ) ;
#8769=VERTEX_POINT ( 'NONE', #13806 ) ;
#8791=FACE_OUTER_BOUND ( 'NONE', #44094, .T. ) ;
#8857=EDGE_CURVE ( 'NONE', #17019, #21881, #70952, .T. ) ;
#8862=VECTOR ( 'NONE', #44359, 1000.000000000000000 ) ;
#8902=EDGE_LOOP ( 'NONE', ( #61469, #24181, #17598, #56020 ) ) ;
#8917=ORIENTED_EDGE ( 'NONE', *, *, #16462, .T. ) ;
#8921=CARTESIAN_POINT ( 'NONE',  ( 19.12409105625796357, -101.5943176906707919, -2.500000000000000000 ) ) ;
#8927=CARTESIAN_POINT ( 'NONE',  ( 3.429551818649054340, -146.3199197248623875, -5.500000000000000000 ) ) ;
#8953=CARTESIAN_POINT ( 'NONE',  ( -6.880223345695647197, -142.5202692415819854, 5.500000000000000000 ) ) ;
#8972=LINE ( 'NONE', #66497, #29858 ) ;
#8983=FACE_BOUND ( 'NONE', #3745, .T. ) ;
#9024=DIRECTION ( 'NONE',  ( -0.000000000000000000, -0.000000000000000000, 1.000000000000000000 ) ) ;
#9028=VECTOR ( 'NONE', #22208, 1000.000000000000000 ) ;
#9046=FACE_BOUND ( 'NONE', #55309, .T. ) ;
#9049=ORIENTED_EDGE ( 'NONE', *, *, #7869, .T. ) ;
#9052=FACE_OUTER_BOUND ( 'NONE', #3794, .T. ) ;
#9073=PLANE ( 'NONE',  #72090 ) ;
#9083=LINE ( 'NONE', #25638, #51803 ) ;
#9102=DIRECTION ( 'NONE',  ( 0.9827303690289279636, 0.1850432970638682395, 0.000000000000000000 ) ) ;
#9120=DIRECTION ( 'NONE',  ( -0.9781476007338042455, -0.2079116908177664758, 0.000000000000000000 ) ) ;
#9134=VERTEX_POINT ( 'NONE', #29164 ) ;
#9137=AXIS2_PLACEMENT_3D ( 'NONE', #33608, #61827, #4696 ) ;
#9140=CARTESIAN_POINT ( 'NONE',  ( -22.53294031248082163, -134.0273518838794757, -5.500000000000000000 ) ) ;
#9159=VECTOR ( 'NONE', #70324, 1000.000000000000000 ) ;
#9168=UNCERTAINTY_MEASURE_WITH_UNIT (LENGTH_MEASURE( 1.000000000000000082E-05 ), #64422, 'distance_accuracy_value', 'NONE');
#9171=ORIENTED_EDGE ( 'NONE', *, *, #2505, .T. ) ;
#9173=EDGE_CURVE ( 'NONE', #46172, #43278, #52105, .T. ) ;
#9176=CARTESIAN_POINT ( 'NONE',  ( 0.000000000000000000, -120.0000000000000000, -5.500000000000000000 ) ) ;
#9182=VECTOR ( 'NONE', #43584, 1000.000000000000000 ) ;
#9192=PLANE ( 'NONE',  #31127 ) ;
#9193=EDGE_CURVE ( 'NONE', #28941, #40320, #23181, .T. ) ;
#9203=VECTOR ( 'NONE', #21391, 1000.000000000000000 ) ;
#9231=VECTOR ( 'NONE', #23620, 999.9999999999998863 ) ;
#9252=DIRECTION ( 'NONE',  ( -0.000000000000000000, -0.000000000000000000, -1.000000000000000000 ) ) ;
#9253=EDGE_CURVE ( 'NONE', #14738, #49489, #14451, .T. ) ;
#9261=AXIS2_PLACEMENT_3D ( 'NONE', #34184, #67659, #39465 ) ;
#9270=EDGE_LOOP ( 'NONE', ( #43216, #60796, #43750, #52706 ) ) ;
#9311=VERTEX_POINT ( 'NONE', #64142 ) ;
#9320=EDGE_LOOP ( 'NONE', ( #51600, #69077, #38006, #28204 ) ) ;
#9346=CARTESIAN_POINT ( 'NONE',  ( 24.95699195200416654, -110.9640411295978595, -5.500000000000000000 ) ) ;
#9358=PLANE ( 'NONE',  #31094 ) ;
#9373=CARTESIAN_POINT ( 'NONE',  ( 16.84844760790522855, -103.5491698323862124, -5.500000000000000000 ) ) ;
#9380=DIRECTION ( 'NONE',  ( -0.6064928550163511956, -0.7950889364178798102, 0.000000000000000000 ) ) ;
#9421=ORIENTED_EDGE ( 'NONE', *, *, #3284, .T. ) ;
#9431=EDGE_LOOP ( 'NONE', ( #38871, #10379, #46703, #69712 ) ) ;
#9451=FACE_OUTER_BOUND ( 'NONE', #50693, .T. ) ;
#9465=LINE ( 'NONE', #21860, #48757 ) ;
#9467=LINE ( 'NONE', #33500, #7049 ) ;
#9487=CARTESIAN_POINT ( 'NONE',  ( -25.50183398199384044, -112.6408924756582053, -2.500000000000000000 ) ) ;
#9497=CARTESIAN_POINT ( 'NONE',  ( 1.384174031800307736, -119.4220188154534981, -2.500000000000000000 ) ) ;
#9517=DIRECTION ( 'NONE',  ( -0.9038112904824853189, 0.4279312458752976833, 0.000000000000000000 ) ) ;
#9525=ORIENTED_EDGE ( 'NONE', *, *, #11894, .F. ) ;
#9533=EDGE_CURVE ( 'NONE', #16806, #23559, #26116, .T. ) ;
#9561=PLANE ( 'NONE',  #45122 ) ;
#9613=AXIS2_PLACEMENT_3D ( 'NONE', #45218, #16261, #23031 ) ;
#9620=EDGE_LOOP ( 'NONE', ( #70267, #23701, #52304, #9833 ) ) ;
#9621=ORIENTED_EDGE ( 'NONE', *, *, #31251, .T. ) ;
#9628=ORIENTED_EDGE ( 'NONE', *, *, #54896, .F. ) ;
#9640=DIRECTION ( 'NONE',  ( -0.1850432970638656582, 0.9827303690289285187, 0.000000000000000000 ) ) ;
#9664=ADVANCED_FACE ( 'NONE', ( #5082 ), #68964, .T. ) ;
#9704=VERTEX_POINT ( 'NONE', #40377 ) ;
#9741=DIRECTION ( 'NONE',  ( 0.9730327541852497042, -0.2306669878475622604, 0.000000000000000000 ) ) ;
#9742=FACE_OUTER_BOUND ( 'NONE', #4874, .T. ) ;
#9754=EDGE_CURVE ( 'NONE', #43361, #30878, #46773, .T. ) ;
#9787=VERTEX_POINT ( 'NONE', #12542 ) ;
#9797=FACE_OUTER_BOUND ( 'NONE', #67470, .T. ) ;
#9812=ORIENTED_EDGE ( 'NONE', *, *, #25825, .F. ) ;
#9833=ORIENTED_EDGE ( 'NONE', *, *, #5881, .T. ) ;
#9840=FACE_OUTER_BOUND ( 'NONE', #39109, .T. ) ;
#9845=VECTOR ( 'NONE', #30601, 1000.000000000000000 ) ;
#9860=CARTESIAN_POINT ( 'NONE',  ( -22.67106064244953245, -113.6342314410295842, 5.500000000000000000 ) ) ;
#9861=EDGE_LOOP ( 'NONE', ( #22424, #70711, #14151, #65268 ) ) ;
#9965=EDGE_LOOP ( 'NONE', ( #57253, #8240, #12675, #58713 ) ) ;
#10000=VECTOR ( 'NONE', #23924, 1000.000000000000000 ) ;
#10024=FACE_OUTER_BOUND ( 'NONE', #2730, .T. ) ;
#10050=VECTOR ( 'NONE', #71239, 1000.000000000000114 ) ;
#10061=DIRECTION ( 'NONE',  ( -0.5687579148473743684, 0.8225049752423791993, 0.000000000000000000 ) ) ;
#10072=LINE ( 'NONE', #66126, #62956 ) ;
#10081=EDGE_LOOP ( 'NONE', ( #31693, #54210, #1625, #72846 ) ) ;
#10085=LINE ( 'NONE', #15346, #9182 ) ;
#10097=VECTOR ( 'NONE', #35765, 1000.000000000000114 ) ;
#10111=CARTESIAN_POINT ( 'NONE',  ( -15.44521549751111422, -137.7748507232956001, 5.500000000000000000 ) ) ;
#10120=DIRECTION ( 'NONE',  ( -0.000000000000000000, -0.000000000000000000, -1.000000000000000000 ) ) ;
#10135=VECTOR ( 'NONE', #19358, 1000.000000000000000 ) ;
#10151=ORIENTED_EDGE ( 'NONE', *, *, #14610, .T. ) ;
#10161=DIRECTION ( 'NONE',  ( 0.9730327541852493711, -0.2306669878475637314, 0.000000000000000000 ) ) ;
#10162=EDGE_CURVE ( 'NONE', #26875, #44562, #54129, .T. ) ;
#10178=CARTESIAN_POINT ( 'NONE',  ( 21.85433023846371370, -135.0628101570779620, 5.500000000000000000 ) ) ;
#10192=ADVANCED_FACE ( 'NONE', ( #4486 ), #9358, .F. ) ;
#10200=VERTEX_POINT ( 'NONE', #32281 ) ;
#10225=VECTOR ( 'NONE', #9640, 1000.000000000000114 ) ;
#10232=ORIENTED_EDGE ( 'NONE', *, *, #53316, .T. ) ;
#10246=CARTESIAN_POINT ( 'NONE',  ( 3.429551818649054340, -146.3199197248623875, 2.500000000000000000 ) ) ;
#10252=ORIENTED_EDGE ( 'NONE', *, *, #13815, .T. ) ;
#10287=EDGE_CURVE ( 'NONE', #33066, #3022, #56811, .T. ) ;
#10293=LINE ( 'NONE', #68181, #73870 ) ;
#10298=ORIENTED_EDGE ( 'NONE', *, *, #51013, .T. ) ;
#10341=ORIENTED_EDGE ( 'NONE', *, *, #13473, .T. ) ;
#10349=PLANE ( 'NONE',  #30935 ) ;
#10353=ORIENTED_EDGE ( 'NONE', *, *, #28330, .F. ) ;
#10379=ORIENTED_EDGE ( 'NONE', *, *, #55741, .F. ) ;
#10384=CARTESIAN_POINT ( 'NONE',  ( -18.12185313557660038, -104.9634299478706794, 5.500000000000000000 ) ) ;
#10391=VECTOR ( 'NONE', #1109, 1000.000000000000000 ) ;
#10409=CARTESIAN_POINT ( 'NONE',  ( 23.41451323550360186, -132.5004227906269989, 5.500000000000000000 ) ) ;
#10422=VECTOR ( 'NONE', #36512, 1000.000000000000000 ) ;
#10432=LINE ( 'NONE', #51774, #19547 ) ;
#10433=DIRECTION ( 'NONE',  ( 0.08130631524010120681, -0.9966891607226784355, 0.000000000000000000 ) ) ;
#10463=LINE ( 'NONE', #62364, #55807 ) ;
#10493=FACE_OUTER_BOUND ( 'NONE', #12187, .T. ) ;
#10528=DIRECTION ( 'NONE',  ( -0.000000000000000000, -0.000000000000000000, 1.000000000000000000 ) ) ;
#10533=ORIENTED_EDGE ( 'NONE', *, *, #3103, .T. ) ;
#10536=EDGE_LOOP ( 'NONE', ( #45213, #29736, #39322, #12549 ) ) ;
#10538=EDGE_CURVE ( 'NONE', #17376, #46993, #66154, .T. ) ;
#10539=ORIENTED_EDGE ( 'NONE', *, *, #60762, .T. ) ;
#10545=ORIENTED_EDGE ( 'NONE', *, *, #50756, .T. ) ;
#10570=DIRECTION ( 'NONE',  ( -0.7950889364178781449, 0.6064928550163533050, 0.000000000000000000 ) ) ;
#10579=VECTOR ( 'NONE', #21684, 1000.000000000000114 ) ;
#10581=DIRECTION ( 'NONE',  ( -0.2306669878475648139, -0.9730327541852491491, 0.000000000000000000 ) ) ;
#10595=EDGE_CURVE ( 'NONE', #37081, #45592, #4485, .T. ) ;
#10596=DIRECTION ( 'NONE',  ( 0.000000000000000000, -0.000000000000000000, 1.000000000000000000 ) ) ;
#10631=DIRECTION ( 'NONE',  ( -0.000000000000000000, -0.000000000000000000, -1.000000000000000000 ) ) ;
#10659=VECTOR ( 'NONE', #2428, 1000.000000000000114 ) ;
#10661=CARTESIAN_POINT ( 'NONE',  ( 23.41451323550362318, -132.5004227906269989, -2.500000000000000000 ) ) ;
#10689=AXIS2_PLACEMENT_3D ( 'NONE', #31272, #36174, #71113 ) ;
#10695=ORIENTED_EDGE ( 'NONE', *, *, #68241, .F. ) ;
#10696=EDGE_CURVE ( 'NONE', #25695, #11562, #11219, .T. ) ;
#10708=CARTESIAN_POINT ( 'NONE',  ( -23.97194136764370498, -131.3950000906648938, 5.500000000000000000 ) ) ;
#10731=ADVANCED_FACE ( 'NONE', ( #481 ), #23251, .F. ) ;
#10760=DIRECTION ( 'NONE',  ( -0.1276937514489679404, -0.9918136447140103451, 0.000000000000000000 ) ) ;
#10780=CARTESIAN_POINT ( 'NONE',  ( -24.50849501662245800, -109.8101191361138831, 5.500000000000000000 ) ) ;
#10791=CARTESIAN_POINT ( 'NONE',  ( -70.53423027509626309, -217.0820393249940423, 5.500000000000000000 ) ) ;
#10810=EDGE_LOOP ( 'NONE', ( #11437, #38814, #25531, #66559 ) ) ;
#10814=FACE_OUTER_BOUND ( 'NONE', #44075, .T. ) ;
#10821=CARTESIAN_POINT ( 'NONE',  ( 23.30762065077924916, -123.0008031590507329, 2.500000000000000000 ) ) ;
#10827=VECTOR ( 'NONE', #49671, 1000.000000000000000 ) ;
#10854=CARTESIAN_POINT ( 'NONE',  ( -17.26469406256017791, -140.1601175325492648, -5.500000000000000000 ) ) ;
#10858=ORIENTED_EDGE ( 'NONE', *, *, #23662, .F. ) ;
#10865=PLANE ( 'NONE',  #13969 ) ;
#10872=LINE ( 'NONE', #50336, #43623 ) ;
#10873=CARTESIAN_POINT ( 'NONE',  ( 23.49916127795269460, -121.5130826919798039, 5.500000000000000000 ) ) ;
#10881=EDGE_CURVE ( 'NONE', #42731, #67963, #23992, .T. ) ;
#10891=PLANE ( 'NONE',  #9261 ) ;
#10895=CARTESIAN_POINT ( 'NONE',  ( -10.43921258969510824, -98.89258801967538659, -5.500000000000000000 ) ) ;
#10915=CYLINDRICAL_SURFACE ( 'NONE', #66463, 35.50000000000000711 ) ;
#10949=CARTESIAN_POINT ( 'NONE',  ( -22.53294031248082163, -134.0273518838794757, 5.500000000000000000 ) ) ;
#10981=PLANE ( 'NONE',  #19707 ) ;
#10990=ORIENTED_EDGE ( 'NONE', *, *, #4705, .T. ) ;
#11006=VERTEX_POINT ( 'NONE', #15668 ) ;
#11010=VERTEX_POINT ( 'NONE', #37495 ) ;
#11013=ORIENTED_EDGE ( 'NONE', *, *, #52015, .T. ) ;
#11021=LINE ( 'NONE', #39599, #567 ) ;
#11051=VECTOR ( 'NONE', #16335, 1000.000000000000227 ) ;
#11063=CARTESIAN_POINT ( 'NONE',  ( -12.50000000000000000, -132.5000000000000000, -2.500000000000000000 ) ) ;
#11101=ORIENTED_EDGE ( 'NONE', *, *, #11197, .F. ) ;
#11104=CARTESIAN_POINT ( 'NONE',  ( -19.27444613274700913, -101.8135840178490668, -2.500000000000000000 ) ) ;
#11143=ORIENTED_EDGE ( 'NONE', *, *, #36952, .T. ) ;
#11147=VECTOR ( 'NONE', #23083, 1000.000000000000000 ) ;
#11159=EDGE_CURVE ( 'NONE', #12862, #42731, #45742, .T. ) ;
#11162=LINE ( 'NONE', #62691, #14571 ) ;
#11175=EDGE_LOOP ( 'NONE', ( #43372, #22746, #15529, #54203 ) ) ;
#11197=EDGE_CURVE ( 'NONE', #34299, #3022, #50985, .T. ) ;
#11210=FACE_OUTER_BOUND ( 'NONE', #16939, .T. ) ;
#11219=LINE ( 'NONE', #10854, #19126 ) ;
#11289=AXIS2_PLACEMENT_3D ( 'NONE', #37789, #53585, #14472 ) ;
#11307=VERTEX_POINT ( 'NONE', #35174 ) ;
#11337=PLANE ( 'NONE',  #49755 ) ;
#11340=AXIS2_PLACEMENT_3D ( 'NONE', #58304, #7175, #31201 ) ;
#11345=EDGE_LOOP ( 'NONE', ( #40339, #8128, #26990, #1723 ) ) ;
#11355=VERTEX_POINT ( 'NONE', #6252 ) ;
#11364=ORIENTED_EDGE ( 'NONE', *, *, #17720, .T. ) ;
#11381=DIRECTION ( 'NONE',  ( -0.000000000000000000, -0.000000000000000000, -1.000000000000000000 ) ) ;
#11389=ORIENTED_EDGE ( 'NONE', *, *, #6525, .F. ) ;
#11406=EDGE_LOOP ( 'NONE', ( #38025, #56497, #22933, #69550 ) ) ;
#11434=ADVANCED_FACE ( 'NONE', ( #25288 ), #31649, .F. ) ;
#11437=ORIENTED_EDGE ( 'NONE', *, *, #49071, .F. ) ;
#11485=CARTESIAN_POINT ( 'NONE',  ( 4.903647372192503795, -146.0423547792665886, 2.500000000000000000 ) ) ;
#11497=DIRECTION ( 'NONE',  ( -0.1276937514489679404, -0.9918136447140103451, 0.000000000000000000 ) ) ;
#11510=PLANE ( 'NONE',  #24122 ) ;
#11558=ADVANCED_FACE ( 'NONE', ( #33126 ), #38039, .F. ) ;
#11562=VERTEX_POINT ( 'NONE', #66616 ) ;
#11617=EDGE_LOOP ( 'NONE', ( #7884, #69963, #23591, #45824 ) ) ;
#11636=PLANE ( 'NONE',  #55714 ) ;
#11655=CIRCLE ( 'NONE', #8075, 35.50000000000000711 ) ;
#11659=ORIENTED_EDGE ( 'NONE', *, *, #71967, .F. ) ;
#11673=VECTOR ( 'NONE', #66753, 1000.000000000000114 ) ;
#11676=VECTOR ( 'NONE', #70627, 1000.000000000000227 ) ;
#11692=ADVANCED_FACE ( 'NONE', ( #52650 ), #28599, .T. ) ;
#11708=ORIENTED_EDGE ( 'NONE', *, *, #39297, .T. ) ;
#11723=VERTEX_POINT ( 'NONE', #65427 ) ;
#11728=VECTOR ( 'NONE', #73744, 1000.000000000000000 ) ;
#11741=DIRECTION ( 'NONE',  ( -0.7950889364178796992, 0.6064928550163511956, 0.000000000000000000 ) ) ;
#11768=DIRECTION ( 'NONE',  ( -0.6064928550163533050, -0.7950889364178781449, 0.000000000000000000 ) ) ;
#11796=ORIENTED_EDGE ( 'NONE', *, *, #16762, .F. ) ;
#11850=CARTESIAN_POINT ( 'NONE',  ( 19.12409105625795291, -101.5943176906707919, 5.500000000000000000 ) ) ;
#11853=ORIENTED_EDGE ( 'NONE', *, *, #45769, .F. ) ;
#11874=CARTESIAN_POINT ( 'NONE',  ( 15.07208474345548055, -141.7963818439230010, -2.500000000000000000 ) ) ;
#11875=DIRECTION ( 'NONE',  ( 1.000000000000000000, 0.000000000000000000, 0.000000000000000000 ) ) ;
#11879=EDGE_CURVE ( 'NONE', #71554, #43361, #32291, .T. ) ;
#11894=EDGE_CURVE ( 'NONE', #70823, #8033, #55979, .T. ) ;
#11932=LINE ( 'NONE', #5582, #55419 ) ;
#11947=VERTEX_POINT ( 'NONE', #3034 ) ;
#11973=DIRECTION ( 'NONE',  ( 1.000000000000000000, 0.000000000000000000, 0.000000000000000000 ) ) ;
#12025=ORIENTED_EDGE ( 'NONE', *, *, #60638, .F. ) ;
#12043=EDGE_LOOP ( 'NONE', ( #55470, #29108, #10545, #73290 ) ) ;
#12071=CARTESIAN_POINT ( 'NONE',  ( -13.05994868825747446, -139.5943292883446532, -2.500000000000000000 ) ) ;
#12079=VERTEX_POINT ( 'NONE', #70949 ) ;
#12081=PLANE ( 'NONE',  #13078 ) ;
#12085=AXIS2_PLACEMENT_3D ( 'NONE', #22058, #51001, #11875 ) ;
#12090=SURFACE_SIDE_STYLE ('',( #41407 ) ) ;
#12111=ORIENTED_EDGE ( 'NONE', *, *, #41841, .F. ) ;
#12113=ORIENTED_EDGE ( 'NONE', *, *, #11197, .T. ) ;
#12120=CARTESIAN_POINT ( 'NONE',  ( -23.54415474984308787, -120.4156646670583086, 5.500000000000000000 ) ) ;
#12123=ADVANCED_FACE ( 'NONE', ( #1842 ), #19083, .F. ) ;
#12142=VERTEX_POINT ( 'NONE', #70567 ) ;
#12159=DIRECTION ( 'NONE',  ( -0.4279312458752990711, -0.9038112904824846527, 0.000000000000000000 ) ) ;
#12161=DIRECTION ( 'NONE',  ( 0.7273375899149793211, -0.6862798483830554463, 0.000000000000000000 ) ) ;
#12165=PLANE ( 'NONE',  #42061 ) ;
#12167=VECTOR ( 'NONE', #66550, 1000.000000000000000 ) ;
#12183=AXIS2_PLACEMENT_3D ( 'NONE', #3836, #49664, #50413 ) ;
#12187=EDGE_LOOP ( 'NONE', ( #67244, #67704, #24399, #63357 ) ) ;
#12201=DIRECTION ( 'NONE',  ( 0.6862798483830533369, 0.7273375899149812085, -0.000000000000000000 ) ) ;
#12223=VERTEX_POINT ( 'NONE', #8921 ) ;
#12248=DIRECTION ( 'NONE',  ( 1.000000000000000000, 0.000000000000000000, 0.000000000000000000 ) ) ;
#12274=ORIENTED_EDGE ( 'NONE', *, *, #61713, .F. ) ;
#12315=ORIENTED_EDGE ( 'NONE', *, *, #34357, .T. ) ;
#12346=CARTESIAN_POINT ( 'NONE',  ( -10.43921258969510824, -98.89258801967538659, 5.500000000000000000 ) ) ;
#12350=VECTOR ( 'NONE', #39665, 999.9999999999998863 ) ;
#12402=ORIENTED_EDGE ( 'NONE', *, *, #10162, .T. ) ;
#12455=( LENGTH_UNIT ( ) NAMED_UNIT ( * ) SI_UNIT ( .MILLI., .METRE. ) );
#12504=LINE ( 'NONE', #35440, #28986 ) ;
#12524=CARTESIAN_POINT ( 'NONE',  ( -21.33958957442910886, -129.9559990355020034, 5.500000000000000000 ) ) ;
#12528=CARTESIAN_POINT ( 'NONE',  ( 0.000000000000000000, -120.0000000000000000, -2.500000000000000000 ) ) ;
#12531=CARTESIAN_POINT ( 'NONE',  ( 12.69589495141918611, -96.69089767102708777, 5.500000000000000000 ) ) ;
#12533=SURFACE_STYLE_USAGE ( .BOTH. , #47854 ) ;
#12542=CARTESIAN_POINT ( 'NONE',  ( -16.06301359042743115, -102.7814171781257357, -5.500000000000000000 ) ) ;
#12549=ORIENTED_EDGE ( 'NONE', *, *, #64209, .T. ) ;
#12551=ORIENTED_EDGE ( 'NONE', *, *, #48136, .F. ) ;
#12559=AXIS2_PLACEMENT_3D ( 'NONE', #19867, #8606, #2990 ) ;
#12563=CARTESIAN_POINT ( 'NONE',  ( 19.12409105625795291, -101.5943176906707919, -5.500000000000000000 ) ) ;
#12588=CARTESIAN_POINT ( 'NONE',  ( -7.572224309238338336, -145.4393675041377492, 2.500000000000000000 ) ) ;
#12641=FACE_OUTER_BOUND ( 'NONE', #50822, .T. ) ;
#12642=VECTOR ( 'NONE', #4324, 1000.000000000000000 ) ;
#12645=EDGE_CURVE ( 'NONE', #34836, #11723, #49424, .T. ) ;
#12660=EDGE_CURVE ( 'NONE', #31608, #9704, #61457, .T. ) ;
#12675=ORIENTED_EDGE ( 'NONE', *, *, #51193, .T. ) ;
#12678=CARTESIAN_POINT ( 'NONE',  ( 26.47460221209471598, -121.8961639463267090, 5.500000000000000000 ) ) ;
#12692=VERTEX_POINT ( 'NONE', #62195 ) ;
#12695=PLANE ( 'NONE',  #24916 ) ;
#12699=AXIS2_PLACEMENT_3D ( 'NONE', #33636, #58053, #46043 ) ;
#12707=DIRECTION ( 'NONE',  ( -0.1850432970638667129, 0.9827303690289281857, 0.000000000000000000 ) ) ;
#12708=DIRECTION ( 'NONE',  ( 0.4796670183876317051, -0.8774505977381972244, 0.000000000000000000 ) ) ;
#12712=CARTESIAN_POINT ( 'NONE',  ( -48.80839716909612491, -10.37454508288793065, 5.500000000000000000 ) ) ;
#12715=ADVANCED_FACE ( 'NONE', ( #63314 ), #34351, .T. ) ;
#12726=AXIS2_PLACEMENT_3D ( 'NONE', #35395, #47056, #41046 ) ;
#12745=EDGE_CURVE ( 'NONE', #56693, #44676, #50534, .T. ) ;
#12748=DIRECTION ( 'NONE',  ( -0.4279312458752977388, -0.9038112904824853189, 0.000000000000000000 ) ) ;
#12818=DIRECTION ( 'NONE',  ( 0.5200609990132993854, 0.8541291221503274356, 0.000000000000000000 ) ) ;
#12862=VERTEX_POINT ( 'NONE', #52380 ) ;
#12879=LINE ( 'NONE', #63301, #24721 ) ;
#12920=ORIENTED_EDGE ( 'NONE', *, *, #64847, .F. ) ;
#12966=CIRCLE ( 'NONE', #14141, 35.50000000000000711 ) ;
#12980=CARTESIAN_POINT ( 'NONE',  ( 19.12409105625795291, -101.5943176906707919, 5.500000000000000000 ) ) ;
#12997=EDGE_CURVE ( 'NONE', #61868, #53859, #30188, .T. ) ;
#13008=CYLINDRICAL_SURFACE ( 'NONE', #73850, 35.50000000000000711 ) ;
#13013=CARTESIAN_POINT ( 'NONE',  ( 21.07894319797337701, -103.8699611390234878, 5.500000000000000000 ) ) ;
#13018=DIRECTION ( 'NONE',  ( -0.1850432970638667129, 0.9827303690289281857, 0.000000000000000000 ) ) ;
#13020=LINE ( 'NONE', #58155, #5805 ) ;
#13043=VECTOR ( 'NONE', #18359, 1000.000000000000114 ) ;
#13045=LINE ( 'NONE', #36352, #5374 ) ;
#13053=ADVANCED_FACE ( 'NONE', ( #25303, #8748 ), #8002, .F. ) ;
#13078=AXIS2_PLACEMENT_3D ( 'NONE', #34267, #45198, #68869 ) ;
#13080=CARTESIAN_POINT ( 'NONE',  ( 19.29194287201271862, -133.5026271600380880, 5.500000000000000000 ) ) ;
#13087=CARTESIAN_POINT ( 'NONE',  ( -9.055038557894883766, -98.31460683512894150, 2.500000000000000000 ) ) ;
#13112=CARTESIAN_POINT ( 'NONE',  ( -26.29030328629083968, -123.6496510949466341, 5.500000000000000000 ) ) ;
#13114=ORIENTED_EDGE ( 'NONE', *, *, #62936, .F. ) ;
#13123=VECTOR ( 'NONE', #17636, 1000.000000000000000 ) ;
#13135=FACE_BOUND ( 'NONE', #22881, .T. ) ;
#13148=ORIENTED_EDGE ( 'NONE', *, *, #52870, .F. ) ;
#13157=FACE_OUTER_BOUND ( 'NONE', #62614, .T. ) ;
#13171=CARTESIAN_POINT ( 'NONE',  ( 16.30584220631899228, -140.9432449716519784, -2.500000000000000000 ) ) ;
#13206=ORIENTED_EDGE ( 'NONE', *, *, #30615, .T. ) ;
#13222=ORIENTED_EDGE ( 'NONE', *, *, #51624, .T. ) ;
#13230=PLANE ( 'NONE',  #67674 ) ;
#13308=LINE ( 'NONE', #1707, #46475 ) ;
#13324=CARTESIAN_POINT ( 'NONE',  ( -6.880223345695647197, -142.5202692415819854, -5.500000000000000000 ) ) ;
#13363=LINE ( 'NONE', #24649, #54463 ) ;
#13371=VECTOR ( 'NONE', #23427, 1000.000000000000114 ) ;
#13381=ORIENTED_EDGE ( 'NONE', *, *, #69082, .F. ) ;
#13401=ORIENTED_EDGE ( 'NONE', *, *, #61612, .T. ) ;
#13409=LINE ( 'NONE', #2175, #2332 ) ;
#13418=EDGE_CURVE ( 'NONE', #43453, #55469, #18934, .T. ) ;
#13464=ORIENTED_EDGE ( 'NONE', *, *, #31251, .F. ) ;
#13473=EDGE_CURVE ( 'NONE', #6773, #57738, #1340, .T. ) ;
#13500=ORIENTED_EDGE ( 'NONE', *, *, #18270, .T. ) ;
#13502=DIRECTION ( 'NONE',  ( -0.000000000000000000, -0.000000000000000000, -1.000000000000000000 ) ) ;
#13536=CARTESIAN_POINT ( 'NONE',  ( 2.874421927457452952, -143.3717286177755739, 5.500000000000000000 ) ) ;
#13538=CARTESIAN_POINT ( 'NONE',  ( 18.80329974962065265, -105.8248132807389084, -5.500000000000000000 ) ) ;
#13541=DIRECTION ( 'NONE',  ( 0.02332147558787931590, 0.9997280174009348652, -0.000000000000000000 ) ) ;
#13562=FILL_AREA_STYLE ('',( #41770 ) ) ;
#13599=CARTESIAN_POINT ( 'NONE',  ( -0.8815729230226008184, -93.47222532549339746, 2.500000000000000000 ) ) ;
#13625=CARTESIAN_POINT ( 'NONE',  ( -12.50000000000000000, -107.5000000000000000, 2.500000000000000000 ) ) ;
#13635=DIRECTION ( 'NONE',  ( -0.000000000000000000, -0.000000000000000000, -1.000000000000000000 ) ) ;
#13661=CARTESIAN_POINT ( 'NONE',  ( 32.50000000000000000, -120.0000000000000000, -2.500000000000000000 ) ) ;
#13662=ORIENTED_EDGE ( 'NONE', *, *, #7664, .F. ) ;
#13663=AXIS2_PLACEMENT_3D ( 'NONE', #35980, #29584, #19058 ) ;
#13677=VERTEX_POINT ( 'NONE', #9140 ) ;
#13700=FACE_OUTER_BOUND ( 'NONE', #1343, .T. ) ;
#13704=CARTESIAN_POINT ( 'NONE',  ( -0.8815729230226008184, -93.47222532549339746, 5.500000000000000000 ) ) ;
#13708=ORIENTED_EDGE ( 'NONE', *, *, #18464, .T. ) ;
#13726=DIRECTION ( 'NONE',  ( 0.5200609990133008287, 0.8541291221503266584, -0.000000000000000000 ) ) ;
#13739=AXIS2_PLACEMENT_3D ( 'NONE', #70622, #59367, #46607 ) ;
#13744=VECTOR ( 'NONE', #26036, 1000.000000000000114 ) ;
#13746=ORIENTED_EDGE ( 'NONE', *, *, #2671, .T. ) ;
#13752=CARTESIAN_POINT ( 'NONE',  ( 2.874421927457452952, -143.3717286177755739, 5.500000000000000000 ) ) ;
#13782=CARTESIAN_POINT ( 'NONE',  ( -16.06301359042743115, -102.7814171781257357, 5.500000000000000000 ) ) ;
#13787=CARTESIAN_POINT ( 'NONE',  ( -0.9515373497862389396, -96.47140937769621871, 2.500000000000000000 ) ) ;
#13788=VECTOR ( 'NONE', #15998, 1000.000000000000000 ) ;
#13806=CARTESIAN_POINT ( 'NONE',  ( 35.50000000000000711, -120.0000000000000000, -5.500000000000000000 ) ) ;
#13808=LINE ( 'NONE', #18347, #4879 ) ;
#13812=DIRECTION ( 'NONE',  ( -0.000000000000000000, -0.000000000000000000, -1.000000000000000000 ) ) ;
#13813=CARTESIAN_POINT ( 'NONE',  ( -18.24502636017238899, -100.7225776329765665, -5.500000000000000000 ) ) ;
#13815=EDGE_CURVE ( 'NONE', #51420, #26020, #61402, .T. ) ;
#13816=PLANE ( 'NONE',  #6122 ) ;
#13835=ADVANCED_FACE ( 'NONE', ( #68146 ), #56123, .F. ) ;
#13838=VECTOR ( 'NONE', #27533, 1000.000000000000000 ) ;
#13844=ORIENTED_EDGE ( 'NONE', *, *, #30619, .F. ) ;
#13847=CARTESIAN_POINT ( 'NONE',  ( -14.87942725330654348, -141.9795960975983178, 5.500000000000000000 ) ) ;
#13851=FACE_OUTER_BOUND ( 'NONE', #3210, .T. ) ;
#13866=DIRECTION ( 'NONE',  ( 0.4279312458752991266, 0.9038112904824847638, 0.000000000000000000 ) ) ;
#13876=EDGE_LOOP ( 'NONE', ( #30396, #49612 ) ) ;
#13889=LINE ( 'NONE', #59778, #37973 ) ;
#13926=ORIENTED_EDGE ( 'NONE', *, *, #24041, .T. ) ;
#13934=FACE_BOUND ( 'NONE', #48832, .T. ) ;
#13943=ORIENTED_EDGE ( 'NONE', *, *, #33731, .T. ) ;
#13952=FACE_OUTER_BOUND ( 'NONE', #17844, .T. ) ;
#13957=VERTEX_POINT ( 'NONE', #57977 ) ;
#13969=AXIS2_PLACEMENT_3D ( 'NONE', #22521, #73259, #15758 ) ;
#14025=VERTEX_POINT ( 'NONE', #65840 ) ;
#14045=ORIENTED_EDGE ( 'NONE', *, *, #5644, .T. ) ;
#14084=EDGE_CURVE ( 'NONE', #12862, #12692, #54551, .T. ) ;
#14086=FACE_OUTER_BOUND ( 'NONE', #32611, .T. ) ;
#14094=EDGE_CURVE ( 'NONE', #14025, #28347, #48540, .T. ) ;
#14115=VECTOR ( 'NONE', #32400, 1000.000000000000114 ) ;
#14141=AXIS2_PLACEMENT_3D ( 'NONE', #12528, #35464, #6892 ) ;
#14146=CARTESIAN_POINT ( 'NONE',  ( -8.826826895187510402, -94.96827758698185562, -5.500000000000000000 ) ) ;
#14151=ORIENTED_EDGE ( 'NONE', *, *, #42274, .F. ) ;
#14155=EDGE_CURVE ( 'NONE', #31529, #28408, #21067, .T. ) ;
#14169=ORIENTED_EDGE ( 'NONE', *, *, #44246, .F. ) ;
#14188=EDGE_CURVE ( 'NONE', #56042, #36390, #27074, .T. ) ;
#14195=DIRECTION ( 'NONE',  ( -0.6064928550163524168, -0.7950889364178789220, 0.000000000000000000 ) ) ;
#14197=VECTOR ( 'NONE', #43862, 1000.000000000000000 ) ;
#14203=CARTESIAN_POINT ( 'NONE',  ( 26.09152095774781799, -124.8716048804687375, 5.500000000000000000 ) ) ;
#14218=ORIENTED_EDGE ( 'NONE', *, *, #54821, .F. ) ;
#14221=VERTEX_POINT ( 'NONE', #44018 ) ;
#14246=FACE_BOUND ( 'NONE', #32230, .T. ) ;
#14247=EDGE_LOOP ( 'NONE', ( #5910, #53992, #17097, #67385 ) ) ;
#14259=CARTESIAN_POINT ( 'NONE',  ( -18.12185313557660038, -104.9634299478706794, 5.500000000000000000 ) ) ;
#14266=DIRECTION ( 'NONE',  ( -0.000000000000000000, -0.000000000000000000, -1.000000000000000000 ) ) ;
#14280=DIRECTION ( 'NONE',  ( -0.000000000000000000, -0.000000000000000000, -1.000000000000000000 ) ) ;
#14297=FACE_OUTER_BOUND ( 'NONE', #11617, .T. ) ;
#14335=ADVANCED_FACE ( 'NONE', ( #71 ), #18406, .F. ) ;
#14336=VECTOR ( 'NONE', #48202, 1000.000000000000000 ) ;
#14340=FACE_OUTER_BOUND ( 'NONE', #52591, .T. ) ;
#14342=EDGE_LOOP ( 'NONE', ( #5008, #60947, #43654, #14045 ) ) ;
#14348=PLANE ( 'NONE',  #34733 ) ;
#14365=CARTESIAN_POINT ( 'NONE',  ( 12.69589495141918611, -96.69089767102708777, 5.500000000000000000 ) ) ;
#14451=CIRCLE ( 'NONE', #15635, 35.50000000000000711 ) ;
#14458=CARTESIAN_POINT ( 'NONE',  ( 114.1267819554180392, -82.91796067500511924, 5.500000000000000000 ) ) ;
#14465=AXIS2_PLACEMENT_3D ( 'NONE', #29152, #46458, #47837 ) ;
#14472=DIRECTION ( 'NONE',  ( 0.4796670183876317051, -0.8774505977381971134, 0.000000000000000000 ) ) ;
#14498=LINE ( 'NONE', #47986, #48420 ) ;
#14516=DIRECTION ( 'NONE',  ( 0.5687579148473752566, -0.8225049752423786442, 0.000000000000000000 ) ) ;
#14518=ADVANCED_FACE ( 'NONE', ( #71747 ), #59383, .F. ) ;
#14523=ADVANCED_FACE ( 'NONE', ( #20252, #7871, #31908, #65404, #30788, #8238, #59018, #70636, #14246, #8983, #7511, #1908, #13135, #71012, #41712, #54845, #24792 ), #42464, .F. ) ;
#14531=CARTESIAN_POINT ( 'NONE',  ( 26.09152095774781799, -124.8716048804687375, 5.500000000000000000 ) ) ;
#14541=EDGE_LOOP ( 'NONE', ( #13662, #68437, #51240, #17508 ) ) ;
#14566=EDGE_LOOP ( 'NONE', ( #58695, #27286 ) ) ;
#14571=VECTOR ( 'NONE', #73933, 1000.000000000000114 ) ;
#14584=EDGE_LOOP ( 'NONE', ( #36641, #54995, #32960, #32339 ) ) ;
#14601=LINE ( 'NONE', #72109, #64159 ) ;
#14610=EDGE_CURVE ( 'NONE', #58705, #31970, #39422, .T. ) ;
#14619=ORIENTED_EDGE ( 'NONE', *, *, #2671, .F. ) ;
#14623=VECTOR ( 'NONE', #43857, 1000.000000000000114 ) ;
#14626=LINE ( 'NONE', #38592, #25318 ) ;
#14636=VERTEX_POINT ( 'NONE', #55591 ) ;
#14644=PLANE ( 'NONE',  #32794 ) ;
#14661=ADVANCED_FACE ( 'NONE', ( #61244 ), #21746, .F. ) ;
#14676=DIRECTION ( 'NONE',  ( -0.000000000000000000, -0.000000000000000000, -1.000000000000000000 ) ) ;
#14684=PLANE ( 'NONE',  #41850 ) ;
#14710=VERTEX_POINT ( 'NONE', #9346 ) ;
#14717=VECTOR ( 'NONE', #45787, 1000.000000000000114 ) ;
#14736=DIRECTION ( 'NONE',  ( -0.000000000000000000, -0.000000000000000000, -1.000000000000000000 ) ) ;
#14737=PLANE ( 'NONE',  #35014 ) ;
#14738=VERTEX_POINT ( 'NONE', #6329 ) ;
#14769=AXIS2_PLACEMENT_3D ( 'NONE', #23567, #19029, #20134 ) ;
#14775=VECTOR ( 'NONE', #61631, 1000.000000000000000 ) ;
#14795=EDGE_LOOP ( 'NONE', ( #54233, #68935 ) ) ;
#14816=DIRECTION ( 'NONE',  ( -0.7273375899149812085, 0.6862798483830533369, 0.000000000000000000 ) ) ;
#14818=EDGE_LOOP ( 'NONE', ( #25946, #7494, #11013, #31869 ) ) ;
#14837=AXIS2_PLACEMENT_3D ( 'NONE', #70484, #30281, #58486 ) ;
#14853=ORIENTED_EDGE ( 'NONE', *, *, #68323, .T. ) ;
#14855=CARTESIAN_POINT ( 'NONE',  ( -25.50183398199384754, -112.6408924756582053, -5.500000000000000000 ) ) ;
#14864=CARTESIAN_POINT ( 'NONE',  ( 6.377742925735834234, -145.7647898336708181, -5.500000000000000000 ) ) ;
#14871=ORIENTED_EDGE ( 'NONE', *, *, #8857, .F. ) ;
#14885=ORIENTED_EDGE ( 'NONE', *, *, #22577, .F. ) ;
#14887=EDGE_LOOP ( 'NONE', ( #1059, #37295, #49547, #16345 ) ) ;
#14962=DIRECTION ( 'NONE',  ( 0.2306669878475637314, 0.9730327541852493711, 0.000000000000000000 ) ) ;
#14972=LINE ( 'NONE', #25150, #36982 ) ;
#14992=VERTEX_POINT ( 'NONE', #36355 ) ;
#15008=DIRECTION ( 'NONE',  ( 1.000000000000000000, 0.000000000000000000, -0.000000000000000000 ) ) ;
#15029=EDGE_CURVE ( 'NONE', #49297, #63158, #60785, .T. ) ;
#15044=LINE ( 'NONE', #21050, #28368 ) ;
#15077=FACE_OUTER_BOUND ( 'NONE', #9431, .T. ) ;
#15078=CARTESIAN_POINT ( 'NONE',  ( -0.7195005275814509993, -118.6838241033926948, 2.500000000000000000 ) ) ;
#15084=CARTESIAN_POINT ( 'NONE',  ( -14.87942725330654348, -141.9795960975983178, 5.500000000000000000 ) ) ;
#15116=DIRECTION ( 'NONE',  ( 0.7273375899149793211, -0.6862798483830554463, 0.000000000000000000 ) ) ;
#15124=PLANE ( 'NONE',  #35771 ) ;
#15159=ORIENTED_EDGE ( 'NONE', *, *, #656, .F. ) ;
#15170=CARTESIAN_POINT ( 'NONE',  ( 6.377742925735834234, -145.7647898336708181, 2.500000000000000000 ) ) ;
#15182=DIRECTION ( 'NONE',  ( 0.8225049752423786442, 0.5687579148473752566, -0.000000000000000000 ) ) ;
#15193=DIRECTION ( 'NONE',  ( 0.000000000000000000, 0.000000000000000000, 1.000000000000000000 ) ) ;
#15209=DIRECTION ( 'NONE',  ( -0.000000000000000000, -0.000000000000000000, -1.000000000000000000 ) ) ;
#15226=AXIS2_PLACEMENT_3D ( 'NONE', #8953, #60109, #14962 ) ;
#15249=AXIS2_PLACEMENT_3D ( 'NONE', #27004, #43950, #4861 ) ;
#15260=CARTESIAN_POINT ( 'NONE',  ( 0.000000000000000000, -120.0000000000000000, 2.500000000000000000 ) ) ;
#15272=DIRECTION ( 'NONE',  ( -0.9966891607226786576, -0.08130631524009861166, 0.000000000000000000 ) ) ;
#15276=FACE_OUTER_BOUND ( 'NONE', #70560, .T. ) ;
#15278=DIRECTION ( 'NONE',  ( -0.9038112904824853189, 0.4279312458752977943, 0.000000000000000000 ) ) ;
#15287=EDGE_LOOP ( 'NONE', ( #24801, #19130, #46818, #46117 ) ) ;
#15312=CARTESIAN_POINT ( 'NONE',  ( 21.07894319797337701, -103.8699611390234878, 5.500000000000000000 ) ) ;
#15333=CARTESIAN_POINT ( 'NONE',  ( -23.97194136764370498, -131.3950000906648938, 5.500000000000000000 ) ) ;
#15337=LINE ( 'NONE', #72479, #26938 ) ;
#15346=CARTESIAN_POINT ( 'NONE',  ( 8.700667342345820288, -98.11853780484867116, 5.500000000000000000 ) ) ;
#15363=CARTESIAN_POINT ( 'NONE',  ( -35.50000000000000711, -120.0000000000000000, 2.500000000000000000 ) ) ;
#15406=AXIS2_PLACEMENT_3D ( 'NONE', #10791, #17903, #27705 ) ;
#15423=VERTEX_POINT ( 'NONE', #28838 ) ;
#15428=ORIENTED_EDGE ( 'NONE', *, *, #54846, .F. ) ;
#15430=DIRECTION ( 'NONE',  ( -0.9435911131814395114, 0.3311129884571304971, 0.000000000000000000 ) ) ;
#15464=VECTOR ( 'NONE', #56385, 1000.000000000000000 ) ;
#15466=DIRECTION ( 'NONE',  ( 0.6862798483830534479, 0.7273375899149810975, 0.000000000000000000 ) ) ;
#15492=AXIS2_PLACEMENT_3D ( 'NONE', #45578, #39553, #40287 ) ;
#15500=FACE_BOUND ( 'NONE', #14795, .T. ) ;
#15502=EDGE_CURVE ( 'NONE', #19022, #20908, #33740, .T. ) ;
#15505=EDGE_CURVE ( 'NONE', #7487, #38564, #10432, .T. ) ;
#15529=ORIENTED_EDGE ( 'NONE', *, *, #19028, .F. ) ;
#15533=CARTESIAN_POINT ( 'NONE',  ( 2.874421927457452952, -143.3717286177755739, -5.500000000000000000 ) ) ;
#15548=LINE ( 'NONE', #4661, #58863 ) ;
#15601=VECTOR ( 'NONE', #54060, 1000.000000000000000 ) ;
#15602=VECTOR ( 'NONE', #65127, 1000.000000000000227 ) ;
#15621=CARTESIAN_POINT ( 'NONE',  ( 19.29194287201271862, -133.5026271600380880, 2.500000000000000000 ) ) ;
#15635=AXIS2_PLACEMENT_3D ( 'NONE', #4797, #16420, #39356 ) ;
#15668=CARTESIAN_POINT ( 'NONE',  ( -7.572224309238338336, -145.4393675041377492, 5.500000000000000000 ) ) ;
#15698=DIRECTION ( 'NONE',  ( 0.000000000000000000, 0.000000000000000000, 1.000000000000000000 ) ) ;
#15708=ADVANCED_FACE ( 'NONE', ( #6294 ), #35215, .F. ) ;
#15710=CARTESIAN_POINT ( 'NONE',  ( -1.192633404626841198, -119.0902607174754451, -2.500000000000000000 ) ) ;
#15730=EDGE_CURVE ( 'NONE', #45237, #6205, #42348, .T. ) ;
#15758=DIRECTION ( 'NONE',  ( 0.1276937514489679404, 0.9918136447140103451, 0.000000000000000000 ) ) ;
#15760=VECTOR ( 'NONE', #74186, 1000.000000000000000 ) ;
#15763=CARTESIAN_POINT ( 'NONE',  ( -7.572224309238338336, -145.4393675041377492, 5.500000000000000000 ) ) ;
#15765=DIRECTION ( 'NONE',  ( -0.4279312458752990711, -0.9038112904824846527, 0.000000000000000000 ) ) ;
#15773=EDGE_CURVE ( 'NONE', #21881, #3726, #43477, .T. ) ;
#15774=CARTESIAN_POINT ( 'NONE',  ( 0.9774260708577211521, -121.1378217241763622, -2.500000000000000000 ) ) ;
#15779=EDGE_CURVE ( 'NONE', #71157, #1966, #14498, .T. ) ;
#15786=PLANE ( 'NONE',  #50209 ) ;
#15810=CARTESIAN_POINT ( 'NONE',  ( 18.80329974962065265, -105.8248132807389084, 5.500000000000000000 ) ) ;
#15838=VERTEX_POINT ( 'NONE', #66754 ) ;
#15846=VECTOR ( 'NONE', #72510, 1000.000000000000114 ) ;
#15848=DIRECTION ( 'NONE',  ( 0.8774505977381971134, 0.4796670183876317051, -0.000000000000000000 ) ) ;
#15884=DIRECTION ( 'NONE',  ( 0.7585478161175723821, 0.6516173805718057377, -0.000000000000000000 ) ) ;
#15915=CARTESIAN_POINT ( 'NONE',  ( -1.459549131277904976, -119.6539995182286304, 2.500000000000000000 ) ) ;
#15982=ORIENTED_EDGE ( 'NONE', *, *, #41841, .T. ) ;
#15998=DIRECTION ( 'NONE',  ( -0.000000000000000000, -0.000000000000000000, -1.000000000000000000 ) ) ;
#16001=ORIENTED_EDGE ( 'NONE', *, *, #30803, .T. ) ;
#16009=VERTEX_POINT ( 'NONE', #39302 ) ;
#16021=DIRECTION ( 'NONE',  ( 0.4279312458753000703, 0.9038112904824842087, -0.000000000000000000 ) ) ;
#16025=ORIENTED_EDGE ( 'NONE', *, *, #33334, .F. ) ;
#16037=ADVANCED_FACE ( 'NONE', ( #69976 ), #24146, .F. ) ;
#16038=DIRECTION ( 'NONE',  ( 1.000000000000000000, 0.000000000000000000, 0.000000000000000000 ) ) ;
#16061=EDGE_CURVE ( 'NONE', #60419, #27599, #47794, .T. ) ;
#16086=EDGE_LOOP ( 'NONE', ( #24951, #22707, #12113, #43496 ) ) ;
#16096=CARTESIAN_POINT ( 'NONE',  ( -10.43921258969510824, -98.89258801967538659, 5.500000000000000000 ) ) ;
#16102=ORIENTED_EDGE ( 'NONE', *, *, #7892, .T. ) ;
#16104=FACE_OUTER_BOUND ( 'NONE', #2726, .T. ) ;
#16105=EDGE_CURVE ( 'NONE', #44712, #50088, #41785, .T. ) ;
#16116=EDGE_CURVE ( 'NONE', #11355, #42185, #31242, .T. ) ;
#16143=LINE ( 'NONE', #51094, #58411 ) ;
#16156=CARTESIAN_POINT ( 'NONE',  ( -14.25258209288423750, -138.6845900058201551, 2.500000000000000000 ) ) ;
#16162=FACE_OUTER_BOUND ( 'NONE', #35140, .T. ) ;
#16164=DIRECTION ( 'NONE',  ( -0.4999999999999919509, -0.8660254037844432595, 0.000000000000000000 ) ) ;
#16194=VERTEX_POINT ( 'NONE', #60210 ) ;
#16196=DIRECTION ( 'NONE',  ( -0.9827303690289285187, -0.1850432970638656860, 0.000000000000000000 ) ) ;
#16197=ADVANCED_FACE ( 'NONE', ( #60574 ), #43655, .F. ) ;
#16222=ADVANCED_FACE ( 'NONE', ( #9052 ), #31604, .F. ) ;
#16261=DIRECTION ( 'NONE',  ( 0.000000000000000000, 0.000000000000000000, 1.000000000000000000 ) ) ;
#16303=CARTESIAN_POINT ( 'NONE',  ( -119.3426274441927433, -132.5434155921188619, -5.500000000000000000 ) ) ;
#16309=ORIENTED_EDGE ( 'NONE', *, *, #57724, .T. ) ;
#16313=ADVANCED_FACE ( 'NONE', ( #9797 ), #61675, .F. ) ;
#16318=CARTESIAN_POINT ( 'NONE',  ( 20.85212586905262100, -130.9402397935870965, -5.500000000000000000 ) ) ;
#16323=DIRECTION ( 'NONE',  ( 0.000000000000000000, -0.000000000000000000, 1.000000000000000000 ) ) ;
#16335=DIRECTION ( 'NONE',  ( -0.8541291221503265474, 0.5200609990133007177, 0.000000000000000000 ) ) ;
#16345=ORIENTED_EDGE ( 'NONE', *, *, #43389, .F. ) ;
#16346=AXIS2_PLACEMENT_3D ( 'NONE', #51168, #10570, #62095 ) ;
#16350=CARTESIAN_POINT ( 'NONE',  ( -23.54415474984308787, -120.4156646670583086, 5.500000000000000000 ) ) ;
#16396=CARTESIAN_POINT ( 'NONE',  ( -1.355716935723729089, -119.3581031311870362, 2.500000000000000000 ) ) ;
#16397=LINE ( 'NONE', #10384, #8411 ) ;
#16407=DIRECTION ( 'NONE',  ( -0.000000000000000000, -0.000000000000000000, -1.000000000000000000 ) ) ;
#16414=ADVANCED_FACE ( 'NONE', ( #39115 ), #10915, .T. ) ;
#16420=DIRECTION ( 'NONE',  ( -0.000000000000000000, -0.000000000000000000, 1.000000000000000000 ) ) ;
#16422=FACE_OUTER_BOUND ( 'NONE', #7666, .T. ) ;
#16423=DIRECTION ( 'NONE',  ( 0.08130631524010120681, -0.9966891607226784355, 0.000000000000000000 ) ) ;
#16426=DIRECTION ( 'NONE',  ( 0.3311129884571281101, 0.9435911131814402886, 0.000000000000000000 ) ) ;
#16457=PLANE ( 'NONE',  #63604 ) ;
#16459=ORIENTED_EDGE ( 'NONE', *, *, #55233, .F. ) ;
#16462=EDGE_CURVE ( 'NONE', #70940, #41508, #28556, .T. ) ;
#16473=ORIENTED_EDGE ( 'NONE', *, *, #44973, .T. ) ;
#16507=CARTESIAN_POINT ( 'NONE',  ( 1.355716935723751293, -120.6418968688129496, 2.500000000000000000 ) ) ;
#16510=DIRECTION ( 'NONE',  ( -0.000000000000000000, -0.000000000000000000, -1.000000000000000000 ) ) ;
#16518=VECTOR ( 'NONE', #13502, 1000.000000000000000 ) ;
#16544=FACE_OUTER_BOUND ( 'NONE', #47564, .T. ) ;
#16580=DIRECTION ( 'NONE',  ( -0.9435911131814395114, 0.3311129884571304971, 0.000000000000000000 ) ) ;
#16598=CARTESIAN_POINT ( 'NONE',  ( -12.50000000000000000, -132.5000000000000000, -2.500000000000000000 ) ) ;
#16603=LINE ( 'NONE', #32401, #26782 ) ;
#16607=ADVANCED_FACE ( 'NONE', ( #41333 ), #24406, .F. ) ;
#16628=EDGE_LOOP ( 'NONE', ( #63848, #27149, #48258, #20139 ) ) ;
#16634=DIRECTION ( 'NONE',  ( 0.4796670183876317051, -0.8774505977381971134, 0.000000000000000000 ) ) ;
#16635=ORIENTED_EDGE ( 'NONE', *, *, #56744, .T. ) ;
#16682=LINE ( 'NONE', #27951, #15760 ) ;
#16685=VECTOR ( 'NONE', #5301, 1000.000000000000114 ) ;
#16716=EDGE_CURVE ( 'NONE', #67113, #14221, #10072, .T. ) ;
#16722=EDGE_CURVE ( 'NONE', #27761, #30878, #37180, .T. ) ;
#16729=ORIENTED_EDGE ( 'NONE', *, *, #22042, .F. ) ;
#16753=CARTESIAN_POINT ( 'NONE',  ( 18.80329974962065265, -105.8248132807389084, -2.500000000000000000 ) ) ;
#16762=EDGE_CURVE ( 'NONE', #39126, #35029, #14601, .T. ) ;
#16777=LINE ( 'NONE', #16396, #36139 ) ;
#16778=LINE ( 'NONE', #51342, #38413 ) ;
#16783=DIRECTION ( 'NONE',  ( -0.000000000000000000, -0.000000000000000000, -1.000000000000000000 ) ) ;
#16803=LINE ( 'NONE', #54517, #67005 ) ;
#16806=VERTEX_POINT ( 'NONE', #43573 ) ;
#16868=ORIENTED_EDGE ( 'NONE', *, *, #16105, .T. ) ;
#16889=CARTESIAN_POINT ( 'NONE',  ( -22.67106064244952535, -113.6342314410295842, -2.500000000000000000 ) ) ;
#16893=LINE ( 'NONE', #28522, #51215 ) ;
#16901=AXIS2_PLACEMENT_3D ( 'NONE', #53740, #47730, #25908 ) ;
#16919=LINE ( 'NONE', #5653, #26958 ) ;
#16924=VECTOR ( 'NONE', #29878, 1000.000000000000000 ) ;
#16939=EDGE_LOOP ( 'NONE', ( #54384, #48173, #46378, #22807 ) ) ;
#16956=ORIENTED_EDGE ( 'NONE', *, *, #56209, .T. ) ;
#16959=EDGE_LOOP ( 'NONE', ( #67605, #67320, #25173, #29223 ) ) ;
#17000=EDGE_CURVE ( 'NONE', #33943, #11010, #591, .T. ) ;
#17019=VERTEX_POINT ( 'NONE', #2173 ) ;
#17039=VECTOR ( 'NONE', #5045, 1000.000000000000114 ) ;
#17059=VECTOR ( 'NONE', #39277, 1000.000000000000000 ) ;
#17067=CARTESIAN_POINT ( 'NONE',  ( 0.5480546763151027401, -96.50639159107802811, 2.500000000000000000 ) ) ;
#17097=ORIENTED_EDGE ( 'NONE', *, *, #30803, .F. ) ;
#17214=DIRECTION ( 'NONE',  ( -0.000000000000000000, -0.000000000000000000, -1.000000000000000000 ) ) ;
#17253=LINE ( 'NONE', #56370, #20469 ) ;
#17259=AXIS2_PLACEMENT_3D ( 'NONE', #4547, #10161, #50379 ) ;
#17309=EDGE_LOOP ( 'NONE', ( #22047, #18362, #10695, #36367 ) ) ;
#17335=DIRECTION ( 'NONE',  ( 0.000000000000000000, -1.000000000000000000, 0.000000000000000000 ) ) ;
#17340=ORIENTED_EDGE ( 'NONE', *, *, #28496, .F. ) ;
#17364=FACE_OUTER_BOUND ( 'NONE', #54274, .T. ) ;
#17369=ORIENTED_EDGE ( 'NONE', *, *, #37591, .F. ) ;
#17376=VERTEX_POINT ( 'NONE', #5116 ) ;
#17389=EDGE_CURVE ( 'NONE', #9311, #70940, #56230, .T. ) ;
#17412=VECTOR ( 'NONE', #23686, 1000.000000000000000 ) ;
#17437=DIRECTION ( 'NONE',  ( 1.000000000000000000, 0.000000000000000000, 0.000000000000000000 ) ) ;
#17454=VERTEX_POINT ( 'NONE', #52814 ) ;
#17469=DIRECTION ( 'NONE',  ( -0.7585478161175723821, -0.6516173805718057377, 0.000000000000000000 ) ) ;
#17482=LINE ( 'NONE', #56977, #40696 ) ;
#17488=LINE ( 'NONE', #40052, #64773 ) ;
#17500=DIRECTION ( 'NONE',  ( -0.000000000000000000, -0.000000000000000000, -1.000000000000000000 ) ) ;
#17504=VERTEX_POINT ( 'NONE', #23870 ) ;
#17508=ORIENTED_EDGE ( 'NONE', *, *, #22577, .T. ) ;
#17510=EDGE_CURVE ( 'NONE', #27833, #57544, #29862, .T. ) ;
#17521=DIRECTION ( 'NONE',  ( -0.1276937514489679404, -0.9918136447140103451, 0.000000000000000000 ) ) ;
#17527=CARTESIAN_POINT ( 'NONE',  ( 25.81725066941077529, -113.8380548628854854, 5.500000000000000000 ) ) ;
#17542=ORIENTED_EDGE ( 'NONE', *, *, #41427, .T. ) ;
#17550=FACE_OUTER_BOUND ( 'NONE', #7671, .T. ) ;
#17560=DIRECTION ( 'NONE',  ( -0.000000000000000000, -0.000000000000000000, -1.000000000000000000 ) ) ;
#17579=VECTOR ( 'NONE', #17335, 1000.000000000000000 ) ;
#17598=ORIENTED_EDGE ( 'NONE', *, *, #12997, .F. ) ;
#17636=DIRECTION ( 'NONE',  ( 0.7950889364178796992, -0.6064928550163511956, 0.000000000000000000 ) ) ;
#17662=ORIENTED_EDGE ( 'NONE', *, *, #28608, .T. ) ;
#17686=ORIENTED_EDGE ( 'NONE', *, *, #15502, .T. ) ;
#17717=CYLINDRICAL_SURFACE ( 'NONE', #15492, 35.50000000000000711 ) ;
#17720=EDGE_CURVE ( 'NONE', #36390, #39841, #11021, .T. ) ;
#17746=VECTOR ( 'NONE', #8747, 1000.000000000000000 ) ;
#17761=FACE_OUTER_BOUND ( 'NONE', #66771, .T. ) ;
#17772=AXIS2_PLACEMENT_3D ( 'NONE', #42444, #45420, #21722 ) ;
#17790=CARTESIAN_POINT ( 'NONE',  ( 25.81725066941077529, -113.8380548628854854, 5.500000000000000000 ) ) ;
#17793=DIRECTION ( 'NONE',  ( -0.4999999999999919509, -0.8660254037844432595, 0.000000000000000000 ) ) ;
#17830=ORIENTED_EDGE ( 'NONE', *, *, #25023, .T. ) ;
#17844=EDGE_LOOP ( 'NONE', ( #39959, #63265, #9421, #35864 ) ) ;
#17870=DIRECTION ( 'NONE',  ( 0.3853207896976547087, -0.9227826878668540234, 0.000000000000000000 ) ) ;
#17887=FACE_OUTER_BOUND ( 'NONE', #50852, .T. ) ;
#17895=CARTESIAN_POINT ( 'NONE',  ( 14.59956846177685996, -138.4757300459248484, -5.500000000000000000 ) ) ;
#17903=DIRECTION ( 'NONE',  ( 0.000000000000000000, 0.000000000000000000, 1.000000000000000000 ) ) ;
#17945=LINE ( 'NONE', #69807, #63045 ) ;
#17961=ORIENTED_EDGE ( 'NONE', *, *, #68323, .F. ) ;
#18027=DIRECTION ( 'NONE',  ( 0.1276937514489694392, 0.9918136447140102341, -0.000000000000000000 ) ) ;
#18039=CARTESIAN_POINT ( 'NONE',  ( 19.29194287201271862, -133.5026271600380880, 5.500000000000000000 ) ) ;
#18041=VERTEX_POINT ( 'NONE', #54211 ) ;
#18101=CARTESIAN_POINT ( 'NONE',  ( -17.26469406256017791, -140.1601175325492648, 5.500000000000000000 ) ) ;
#18106=PLANE ( 'NONE',  #12726 ) ;
#18153=VECTOR ( 'NONE', #52439, 1000.000000000000114 ) ;
#18157=VECTOR ( 'NONE', #43972, 1000.000000000000000 ) ;
#18178=CARTESIAN_POINT ( 'NONE',  ( -20.30386590532152979, -102.9045904027214959, 5.500000000000000000 ) ) ;
#18219=VECTOR ( 'NONE', #55697, 999.9999999999998863 ) ;
#18225=CARTESIAN_POINT ( 'NONE',  ( 23.41451323550360186, -132.5004227906269989, 5.500000000000000000 ) ) ;
#18241=EDGE_CURVE ( 'NONE', #15423, #44183, #10463, .T. ) ;
#18266=CARTESIAN_POINT ( 'NONE',  ( 19.12409105625795291, -101.5943176906707919, -5.500000000000000000 ) ) ;
#18270=EDGE_CURVE ( 'NONE', #55143, #73780, #6680, .T. ) ;
#18294=CARTESIAN_POINT ( 'NONE',  ( -23.54415474984308787, -120.4156646670583086, 5.500000000000000000 ) ) ;
#18307=EDGE_CURVE ( 'NONE', #28408, #42171, #13045, .T. ) ;
#18343=DIRECTION ( 'NONE',  ( 0.9966891607226785466, 0.08130631524010119293, -0.000000000000000000 ) ) ;
#18347=CARTESIAN_POINT ( 'NONE',  ( 22.08297821871651934, -111.8242998470044540, 5.500000000000000000 ) ) ;
#18349=CARTESIAN_POINT ( 'NONE',  ( 12.13205353604972991, -140.1820037904669789, 2.500000000000000000 ) ) ;
#18359=DIRECTION ( 'NONE',  ( -0.9580045777625456616, -0.2867529058022021404, 0.000000000000000000 ) ) ;
#18362=ORIENTED_EDGE ( 'NONE', *, *, #53751, .F. ) ;
#18379=EDGE_CURVE ( 'NONE', #35029, #67113, #35251, .T. ) ;
#18406=PLANE ( 'NONE',  #22520 ) ;
#18414=DIRECTION ( 'NONE',  ( -0.000000000000000000, -0.000000000000000000, -1.000000000000000000 ) ) ;
#18451=CARTESIAN_POINT ( 'NONE',  ( 14.59956846177685996, -138.4757300459248484, 5.500000000000000000 ) ) ;
#18461=LINE ( 'NONE', #41405, #31097 ) ;
#18464=EDGE_CURVE ( 'NONE', #65294, #71076, #43129, .T. ) ;
#18481=DIRECTION ( 'NONE',  ( -0.8774505977381983346, -0.4796670183876294291, 0.000000000000000000 ) ) ;
#18483=ORIENTED_EDGE ( 'NONE', *, *, #9754, .T. ) ;
#18516=DIRECTION ( 'NONE',  ( 0.9918136447140101231, -0.1276937514489694114, 0.000000000000000000 ) ) ;
#18535=EDGE_CURVE ( 'NONE', #56042, #10200, #26554, .T. ) ;
#18552=CARTESIAN_POINT ( 'NONE',  ( 21.85433023846371370, -135.0628101570779620, 5.500000000000000000 ) ) ;
#18575=CARTESIAN_POINT ( 'NONE',  ( 22.94323693612312809, -114.6983135802921083, 5.500000000000000000 ) ) ;
#18598=ORIENTED_EDGE ( 'NONE', *, *, #11879, .F. ) ;
#18605=ORIENTED_EDGE ( 'NONE', *, *, #65880, .F. ) ;
#18639=AXIS2_PLACEMENT_3D ( 'NONE', #7065, #1839, #40926 ) ;
#18662=ORIENTED_EDGE ( 'NONE', *, *, #2011, .T. ) ;
#18675=EDGE_LOOP ( 'NONE', ( #44595, #47616, #37190, #11708 ) ) ;
#18692=CARTESIAN_POINT ( 'NONE',  ( -16.06301359042743115, -102.7814171781257357, 5.500000000000000000 ) ) ;
#18700=PLANE ( 'NONE',  #19679 ) ;
#18717=DIRECTION ( 'NONE',  ( -0.000000000000000000, -0.000000000000000000, -1.000000000000000000 ) ) ;
#18721=DIRECTION ( 'NONE',  ( 0.000000000000000000, -0.000000000000000000, 1.000000000000000000 ) ) ;
#18723=LINE ( 'NONE', #13087, #39569 ) ;
#18742=EDGE_LOOP ( 'NONE', ( #23862, #56963, #61412, #28493 ) ) ;
#18743=VECTOR ( 'NONE', #54507, 1000.000000000000000 ) ;
#18789=FACE_OUTER_BOUND ( 'NONE', #14247, .T. ) ;
#18815=EDGE_CURVE ( 'NONE', #52797, #6335, #8069, .T. ) ;
#18843=ORIENTED_EDGE ( 'NONE', *, *, #66224, .F. ) ;
#18850=ORIENTED_EDGE ( 'NONE', *, *, #73188, .F. ) ;
#18853=VECTOR ( 'NONE', #19925, 1000.000000000000000 ) ;
#18934=LINE ( 'NONE', #40398, #64738 ) ;
#18939=LINE ( 'NONE', #10821, #57588 ) ;
#18950=LINE ( 'NONE', #48648, #54711 ) ;
#18979=CARTESIAN_POINT ( 'NONE',  ( 0.1219594728601484379, -121.4950337410840149, -2.500000000000000000 ) ) ;
#18990=CARTESIAN_POINT ( 'NONE',  ( 0.000000000000000000, -120.0000000000000000, 5.500000000000000888 ) ) ;
#18996=DIRECTION ( 'NONE',  ( -0.000000000000000000, -0.000000000000000000, -1.000000000000000000 ) ) ;
#19022=VERTEX_POINT ( 'NONE', #38121 ) ;
#19028=EDGE_CURVE ( 'NONE', #73248, #71157, #37013, .T. ) ;
#19029=DIRECTION ( 'NONE',  ( -0.000000000000000000, -0.000000000000000000, 1.000000000000000000 ) ) ;
#19049=VERTEX_POINT ( 'NONE', #53946 ) ;
#19058=DIRECTION ( 'NONE',  ( -0.5000000000000039968, 0.8660254037844363761, 0.000000000000000000 ) ) ;
#19073=DIRECTION ( 'NONE',  ( -0.000000000000000000, -0.000000000000000000, -1.000000000000000000 ) ) ;
#19083=PLANE ( 'NONE',  #967 ) ;
#19126=VECTOR ( 'NONE', #63124, 1000.000000000000114 ) ;
#19127=VERTEX_POINT ( 'NONE', #28687 ) ;
#19130=ORIENTED_EDGE ( 'NONE', *, *, #73732, .T. ) ;
#19157=EDGE_LOOP ( 'NONE', ( #60200, #56211, #43815, #6386 ) ) ;
#19163=EDGE_LOOP ( 'NONE', ( #53467, #957, #5201, #19891 ) ) ;
#19178=DIRECTION ( 'NONE',  ( -0.000000000000000000, -0.000000000000000000, -1.000000000000000000 ) ) ;
#19196=EDGE_CURVE ( 'NONE', #23559, #24993, #10293, .T. ) ;
#19232=EDGE_LOOP ( 'NONE', ( #17830, #7844 ) ) ;
#19239=CARTESIAN_POINT ( 'NONE',  ( -21.33958957442910886, -129.9559990355020034, 5.500000000000000000 ) ) ;
#19278=CARTESIAN_POINT ( 'NONE',  ( 1.355716935723751293, -120.6418968688129496, -2.500000000000000000 ) ) ;
#19307=EDGE_LOOP ( 'NONE', ( #60935, #44498, #885, #6833 ) ) ;
#19317=VERTEX_POINT ( 'NONE', #41100 ) ;
#19346=ORIENTED_EDGE ( 'NONE', *, *, #12745, .T. ) ;
#19347=DIRECTION ( 'NONE',  ( -0.000000000000000000, -0.000000000000000000, -1.000000000000000000 ) ) ;
#19358=DIRECTION ( 'NONE',  ( -0.000000000000000000, -0.000000000000000000, -1.000000000000000000 ) ) ;
#19378=EDGE_LOOP ( 'NONE', ( #43002, #38947, #66438, #2082 ) ) ;
#19387=AXIS2_PLACEMENT_3D ( 'NONE', #42376, #71667, #49115 ) ;
#19407=EDGE_LOOP ( 'NONE', ( #46223, #33024, #37291, #41105 ) ) ;
#19414=LINE ( 'NONE', #3271, #54633 ) ;
#19429=AXIS2_PLACEMENT_3D ( 'NONE', #71032, #2667, #64669 ) ;
#19444=ADVANCED_FACE ( 'NONE', ( #22937 ), #5284, .F. ) ;
#19456=LINE ( 'NONE', #54053, #29264 ) ;
#19469=DIRECTION ( 'NONE',  ( -0.9227826878668540234, -0.3853207896976547642, 0.000000000000000000 ) ) ;
#19474=CARTESIAN_POINT ( 'NONE',  ( -20.30386590532152979, -102.9045904027214959, 5.500000000000000000 ) ) ;
#19494=PLANE ( 'NONE',  #17772 ) ;
#19501=EDGE_CURVE ( 'NONE', #70242, #61868, #16919, .T. ) ;
#19522=EDGE_CURVE ( 'NONE', #57541, #69025, #24763, .T. ) ;
#19528=CARTESIAN_POINT ( 'NONE',  ( -8.826826895187510402, -94.96827758698185562, -2.500000000000000444 ) ) ;
#19531=CARTESIAN_POINT ( 'NONE',  ( 1.384174031800307736, -119.4220188154534981, 2.500000000000000000 ) ) ;
#19547=VECTOR ( 'NONE', #10061, 1000.000000000000114 ) ;
#19562=DIRECTION ( 'NONE',  ( 0.8225049752423776450, 0.5687579148473765889, 0.000000000000000000 ) ) ;
#19578=FACE_OUTER_BOUND ( 'NONE', #58275, .T. ) ;
#19584=ORIENTED_EDGE ( 'NONE', *, *, #46762, .T. ) ;
#19621=LINE ( 'NONE', #30896, #73954 ) ;
#19679=AXIS2_PLACEMENT_3D ( 'NONE', #726, #41279, #63852 ) ;
#19696=DIRECTION ( 'NONE',  ( 0.8774505977381983346, 0.4796670183876293736, 0.000000000000000000 ) ) ;
#19699=EDGE_CURVE ( 'NONE', #43669, #1173, #72099, .T. ) ;
#19707=AXIS2_PLACEMENT_3D ( 'NONE', #61380, #10596, #4245 ) ;
#19720=DIRECTION ( 'NONE',  ( 0.3090169943749573878, -0.9510565162951503115, 0.000000000000000000 ) ) ;
#19724=LINE ( 'NONE', #8463, #3971 ) ;
#19726=ORIENTED_EDGE ( 'NONE', *, *, #36903, .T. ) ;
#19730=DIRECTION ( 'NONE',  ( 0.9730327541852497042, -0.2306669878475623159, 0.000000000000000000 ) ) ;
#19731=CARTESIAN_POINT ( 'NONE',  ( -3.961125083139900749, -143.2122702051246677, 5.500000000000000000 ) ) ;
#19735=DIRECTION ( 'NONE',  ( 1.000000000000000000, 0.000000000000000000, 0.000000000000000000 ) ) ;
#19787=CARTESIAN_POINT ( 'NONE',  ( 8.700667342345820288, -98.11853780484867116, 5.500000000000000000 ) ) ;
#19794=CARTESIAN_POINT ( 'NONE',  ( -7.670864526094549163, -97.73662565058241114, 5.500000000000000000 ) ) ;
#19822=LINE ( 'NONE', #3311, #46872 ) ;
#19824=LINE ( 'NONE', #42403, #29899 ) ;
#19845=VERTEX_POINT ( 'NONE', #62156 ) ;
#19851=AXIS2_PLACEMENT_3D ( 'NONE', #56114, #67014, #44093 ) ;
#19867=CARTESIAN_POINT ( 'NONE',  ( -17.26469406256017791, -140.1601175325492648, 5.500000000000000000 ) ) ;
#19891=ORIENTED_EDGE ( 'NONE', *, *, #52870, .T. ) ;
#19925=DIRECTION ( 'NONE',  ( -0.8225049752423776450, -0.5687579148473765889, 0.000000000000000000 ) ) ;
#19935=AXIS2_PLACEMENT_3D ( 'NONE', #7195, #63619, #29732 ) ;
#19967=DIRECTION ( 'NONE',  ( -0.9227826878668545785, -0.3853207896976533209, 0.000000000000000000 ) ) ;
#19985=FACE_OUTER_BOUND ( 'NONE', #28500, .T. ) ;
#19988=CARTESIAN_POINT ( 'NONE',  ( -11.59517495878806947, -96.12423995607481686, -5.500000000000000000 ) ) ;
#20002=LINE ( 'NONE', #59140, #30051 ) ;
#20004=FACE_OUTER_BOUND ( 'NONE', #34511, .T. ) ;
#20024=FACE_OUTER_BOUND ( 'NONE', #25869, .T. ) ;
#20032=ADVANCED_FACE ( 'NONE', ( #17761 ), #63650, .F. ) ;
#20038=VECTOR ( 'NONE', #57863, 1000.000000000000000 ) ;
#20051=ORIENTED_EDGE ( 'NONE', *, *, #51102, .T. ) ;
#20064=CARTESIAN_POINT ( 'NONE',  ( 23.11608002360578240, -124.4885236261218182, -2.500000000000000000 ) ) ;
#20073=VERTEX_POINT ( 'NONE', #28294 ) ;
#20079=PLANE ( 'NONE',  #7435 ) ;
#20089=FACE_OUTER_BOUND ( 'NONE', #15287, .T. ) ;
#20099=CARTESIAN_POINT ( 'NONE',  ( -21.33958957442910886, -129.9559990355020034, -5.500000000000000000 ) ) ;
#20130=ORIENTED_EDGE ( 'NONE', *, *, #45584, .F. ) ;
#20131=FACE_OUTER_BOUND ( 'NONE', #49692, .T. ) ;
#20134=DIRECTION ( 'NONE',  ( 1.000000000000000000, 0.000000000000000000, 0.000000000000000000 ) ) ;
#20139=ORIENTED_EDGE ( 'NONE', *, *, #47435, .T. ) ;
#20173=EDGE_CURVE ( 'NONE', #14992, #44417, #38295, .T. ) ;
#20182=ORIENTED_EDGE ( 'NONE', *, *, #62309, .F. ) ;
#20191=FACE_OUTER_BOUND ( 'NONE', #24407, .T. ) ;
#20233=DIRECTION ( 'NONE',  ( -0.000000000000000000, -0.000000000000000000, -1.000000000000000000 ) ) ;
#20252=FACE_BOUND ( 'NONE', #31636, .T. ) ;
#20276=ADVANCED_FACE ( 'NONE', ( #11210 ), #39045, .F. ) ;
#20281=LINE ( 'NONE', #38703, #27983 ) ;
#20297=PLANE ( 'NONE',  #62254 ) ;
#20314=ORIENTED_EDGE ( 'NONE', *, *, #18815, .T. ) ;
#20327=FACE_BOUND ( 'NONE', #36709, .T. ) ;
#20338=ORIENTED_EDGE ( 'NONE', *, *, #62316, .T. ) ;
#20365=ORIENTED_EDGE ( 'NONE', *, *, #9533, .F. ) ;
#20366=DIRECTION ( 'NONE',  ( 0.9227826878668540234, 0.3853207896976547087, 0.000000000000000000 ) ) ;
#20389=ADVANCED_FACE ( 'NONE', ( #16104 ), #58543, .T. ) ;
#20419=CARTESIAN_POINT ( 'NONE',  ( -21.33958957442910886, -129.9559990355020034, 5.500000000000000000 ) ) ;
#20421=CARTESIAN_POINT ( 'NONE',  ( -12.50000000000000000, -132.5000000000000000, 2.500000000000000000 ) ) ;
#20444=PLANE ( 'NONE',  #73087 ) ;
#20462=ORIENTED_EDGE ( 'NONE', *, *, #64847, .T. ) ;
#20469=VECTOR ( 'NONE', #45470, 1000.000000000000000 ) ;
#20480=DIRECTION ( 'NONE',  ( -0.000000000000000000, -0.000000000000000000, -1.000000000000000000 ) ) ;
#20487=AXIS2_PLACEMENT_3D ( 'NONE', #4567, #16196, #3827 ) ;
#20490=VECTOR ( 'NONE', #18414, 1000.000000000000000 ) ;
#20512=VECTOR ( 'NONE', #64505, 1000.000000000000000 ) ;
#20536=VECTOR ( 'NONE', #6359, 1000.000000000000114 ) ;
#20537=DIRECTION ( 'NONE',  ( -0.000000000000000000, -0.000000000000000000, -1.000000000000000000 ) ) ;
#20544=CARTESIAN_POINT ( 'NONE',  ( -0.9774260708577104939, -118.8621782758236378, 2.500000000000000000 ) ) ;
#20564=LINE ( 'NONE', #38600, #70130 ) ;
#20599=ADVANCED_FACE ( 'NONE', ( #37106 ), #31448, .F. ) ;
#20621=PLANE ( 'NONE',  #35379 ) ;
#20646=EDGE_CURVE ( 'NONE', #68795, #43361, #48012, .T. ) ;
#20648=DIRECTION ( 'NONE',  ( -0.6862798483830533369, -0.7273375899149812085, 0.000000000000000000 ) ) ;
#20653=EDGE_CURVE ( 'NONE', #45134, #23125, #54028, .T. ) ;
#20663=LINE ( 'NONE', #3037, #24392 ) ;
#20668=CARTESIAN_POINT ( 'NONE',  ( 24.95699195200416654, -110.9640411295978595, -5.500000000000000000 ) ) ;
#20691=ORIENTED_EDGE ( 'NONE', *, *, #23360, .T. ) ;
#20698=VERTEX_POINT ( 'NONE', #61895 ) ;
#20707=CARTESIAN_POINT ( 'NONE',  ( -0.4966694826856976608, -121.4153866697721611, -2.500000000000000000 ) ) ;
#20722=DIRECTION ( 'NONE',  ( -1.000000000000000000, 0.000000000000000000, -0.000000000000000000 ) ) ;
#20770=LINE ( 'NONE', #32042, #35394 ) ;
#20772=VECTOR ( 'NONE', #49353, 1000.000000000000114 ) ;
#20784=FACE_OUTER_BOUND ( 'NONE', #36547, .T. ) ;
#20789=AXIS2_PLACEMENT_3D ( 'NONE', #73636, #22154, #45094 ) ;
#20795=ORIENTED_EDGE ( 'NONE', *, *, #69620, .T. ) ;
#20800=ADVANCED_FACE ( 'NONE', ( #62268 ), #68652, .F. ) ;
#20804=ORIENTED_EDGE ( 'NONE', *, *, #49134, .F. ) ;
#20825=CARTESIAN_POINT ( 'NONE',  ( 12.13205353604972991, -140.1820037904669789, 5.500000000000000000 ) ) ;
#20841=CARTESIAN_POINT ( 'NONE',  ( 23.11608002360578240, -124.4885236261218182, -5.500000000000000000 ) ) ;
#20846=CARTESIAN_POINT ( 'NONE',  ( -25.50183398199384754, -112.6408924756582053, 5.500000000000000000 ) ) ;
#20851=FACE_OUTER_BOUND ( 'NONE', #38153, .T. ) ;
#20868=ORIENTED_EDGE ( 'NONE', *, *, #37964, .T. ) ;
#20870=LINE ( 'NONE', #55828, #50265 ) ;
#20900=CYLINDRICAL_SURFACE ( 'NONE', #5455, 32.50000000000000000 ) ;
#20907=ADVANCED_FACE ( 'NONE', ( #29880 ), #6600, .F. ) ;
#20908=VERTEX_POINT ( 'NONE', #1372 ) ;
#20913=LINE ( 'NONE', #14531, #21040 ) ;
#20930=EDGE_LOOP ( 'NONE', ( #46676, #58718, #11364, #6973 ) ) ;
#20960=ADVANCED_FACE ( 'NONE', ( #13700 ), #60333, .T. ) ;
#20996=DIRECTION ( 'NONE',  ( -0.9435911131814398445, 0.3311129884571295534, 0.000000000000000000 ) ) ;
#20998=CARTESIAN_POINT ( 'NONE',  ( 17.82587367876289974, -104.6869915565625320, -2.500000000000000000 ) ) ;
#21018=ADVANCED_FACE ( 'NONE', ( #71204 ), #20079, .F. ) ;
#21040=VECTOR ( 'NONE', #32182, 1000.000000000000000 ) ;
#21050=CARTESIAN_POINT ( 'NONE',  ( 6.377742925735834234, -145.7647898336708181, 5.500000000000000000 ) ) ;
#21067=LINE ( 'NONE', #39496, #64480 ) ;
#21080=FACE_OUTER_BOUND ( 'NONE', #37360, .T. ) ;
#21100=EDGE_LOOP ( 'NONE', ( #72123, #61727, #10533, #26807 ) ) ;
#21102=EDGE_CURVE ( 'NONE', #38008, #46917, #50509, .T. ) ;
#21103=AXIS2_PLACEMENT_3D ( 'NONE', #51269, #62580, #17793 ) ;
#21138=DIRECTION ( 'NONE',  ( 0.4796670183876304283, -0.8774505977381978905, 0.000000000000000000 ) ) ;
#21143=ORIENTED_EDGE ( 'NONE', *, *, #66112, .T. ) ;
#21160=PLANE ( 'NONE',  #947 ) ;
#21186=DIRECTION ( 'NONE',  ( -0.9918136447140100120, 0.1276937514489704939, 0.000000000000000000 ) ) ;
#21203=DIRECTION ( 'NONE',  ( 1.000000000000000000, 0.000000000000000000, 0.000000000000000000 ) ) ;
#21244=AXIS2_PLACEMENT_3D ( 'NONE', #25171, #65034, #54473 ) ;
#21257=ORIENTED_EDGE ( 'NONE', *, *, #66224, .T. ) ;
#21274=ADVANCED_FACE ( 'NONE', ( #13157 ), #53027, .F. ) ;
#21290=CARTESIAN_POINT ( 'NONE',  ( -4.653126046682595884, -146.1313684676804314, 5.500000000000000000 ) ) ;
#21300=LINE ( 'NONE', #26950, #15601 ) ;
#21302=DIRECTION ( 'NONE',  ( -0.9997280174009349762, 0.02332147558787671729, 0.000000000000000000 ) ) ;
#21327=CARTESIAN_POINT ( 'NONE',  ( -23.30023580412278505, -123.4057321492263384, 5.500000000000000000 ) ) ;
#21360=VERTEX_POINT ( 'NONE', #73257 ) ;
#21376=VECTOR ( 'NONE', #22198, 1000.000000000000114 ) ;
#21391=DIRECTION ( 'NONE',  ( -0.9227826878668540234, -0.3853207896976546531, 0.000000000000000000 ) ) ;
#21402=DIRECTION ( 'NONE',  ( 0.5687579148473765889, -0.8225049752423776450, 0.000000000000000000 ) ) ;
#21408=VECTOR ( 'NONE', #33715, 1000.000000000000000 ) ;
#21435=LINE ( 'NONE', #61684, #61225 ) ;
#21447=PLANE ( 'NONE',  #20487 ) ;
#21509=CARTESIAN_POINT ( 'NONE',  ( 23.49916127795269460, -121.5130826919798039, 5.500000000000000000 ) ) ;
#21511=ORIENTED_EDGE ( 'NONE', *, *, #38387, .T. ) ;
#21549=VECTOR ( 'NONE', #40952, 1000.000000000000000 ) ;
#21567=ORIENTED_EDGE ( 'NONE', *, *, #30377, .F. ) ;
#21582=VECTOR ( 'NONE', #11768, 1000.000000000000114 ) ;
#21634=FACE_OUTER_BOUND ( 'NONE', #34240, .T. ) ;
#21682=CARTESIAN_POINT ( 'NONE',  ( 0.4966694826857007139, -118.5846133302278247, -2.500000000000000000 ) ) ;
#21684=DIRECTION ( 'NONE',  ( -0.3311129884571280546, -0.9435911131814402886, 0.000000000000000000 ) ) ;
#21694=CARTESIAN_POINT ( 'NONE',  ( 3.429551818649054340, -146.3199197248623875, 5.500000000000000000 ) ) ;
#21701=VECTOR ( 'NONE', #66169, 1000.000000000000114 ) ;
#21722=DIRECTION ( 'NONE',  ( -0.9827303690289279636, -0.1850432970638682117, 0.000000000000000000 ) ) ;
#21724=ORIENTED_EDGE ( 'NONE', *, *, #26062, .T. ) ;
#21746=PLANE ( 'NONE',  #15249 ) ;
#21779=DIRECTION ( 'NONE',  ( 0.8225049752423776450, 0.5687579148473764779, 0.000000000000000000 ) ) ;
#21799=EDGE_CURVE ( 'NONE', #45134, #27007, #5429, .T. ) ;
#21817=AXIS2_PLACEMENT_3D ( 'NONE', #56942, #46031, #73837 ) ;
#21835=ORIENTED_EDGE ( 'NONE', *, *, #63676, .F. ) ;
#21846=PLANE ( 'NONE',  #41027 ) ;
#21860=CARTESIAN_POINT ( 'NONE',  ( -0.9515373497862389396, -96.47140937769621871, 5.500000000000000000 ) ) ;
#21869=LINE ( 'NONE', #66631, #6435 ) ;
#21870=CARTESIAN_POINT ( 'NONE',  ( -24.50849501662245800, -109.8101191361138831, -5.500000000000000000 ) ) ;
#21881=VERTEX_POINT ( 'NONE', #16318 ) ;
#21882=LINE ( 'NONE', #45581, #43777 ) ;
#21898=ORIENTED_EDGE ( 'NONE', *, *, #29375, .T. ) ;
#21927=DIRECTION ( 'NONE',  ( 0.2306669878475637314, 0.9730327541852493711, -0.000000000000000000 ) ) ;
#21951=CARTESIAN_POINT ( 'NONE',  ( -1.474095553543409487, -120.2775649455957989, -2.500000000000000000 ) ) ;
#21958=ORIENTED_EDGE ( 'NONE', *, *, #54155, .F. ) ;
#21980=VECTOR ( 'NONE', #1847, 1000.000000000000114 ) ;
#21987=ADVANCED_FACE ( 'NONE', ( #920 ), #23082, .F. ) ;
#22038=VECTOR ( 'NONE', #62682, 1000.000000000000114 ) ;
#22039=CARTESIAN_POINT ( 'NONE',  ( 26.09152095774781799, -124.8716048804687375, 5.500000000000000000 ) ) ;
#22041=VERTEX_POINT ( 'NONE', #25655 ) ;
#22042=EDGE_CURVE ( 'NONE', #58064, #16194, #59884, .T. ) ;
#22047=ORIENTED_EDGE ( 'NONE', *, *, #54427, .F. ) ;
#22054=PLANE ( 'NONE',  #40441 ) ;
#22058=CARTESIAN_POINT ( 'NONE',  ( 0.000000000000000000, -120.0000000000000000, 2.500000000000000000 ) ) ;
#22077=VECTOR ( 'NONE', #30496, 1000.000000000000000 ) ;
#22094=EDGE_CURVE ( 'NONE', #37728, #13957, #43343, .T. ) ;
#22108=VERTEX_POINT ( 'NONE', #65520 ) ;
#22117=ORIENTED_EDGE ( 'NONE', *, *, #25570, .T. ) ;
#22128=ORIENTED_EDGE ( 'NONE', *, *, #30474, .T. ) ;
#22146=ADVANCED_FACE ( 'NONE', ( #31654 ), #14737, .F. ) ;
#22154=DIRECTION ( 'NONE',  ( 0.1850432970638682395, -0.9827303690289279636, 0.000000000000000000 ) ) ;
#22168=CARTESIAN_POINT ( 'NONE',  ( 11.41210121379328335, -99.40233154247455616, 2.500000000000000000 ) ) ;
#22198=DIRECTION ( 'NONE',  ( 0.9038112904824853189, -0.4279312458752977388, 0.000000000000000000 ) ) ;
#22208=DIRECTION ( 'NONE',  ( 0.5200609990132993854, 0.8541291221503274356, 0.000000000000000000 ) ) ;
#22209=VERTEX_POINT ( 'NONE', #3126 ) ;
#22219=ORIENTED_EDGE ( 'NONE', *, *, #62316, .F. ) ;
#22244=DIRECTION ( 'NONE',  ( -0.000000000000000000, -0.000000000000000000, -1.000000000000000000 ) ) ;
#22247=CARTESIAN_POINT ( 'NONE',  ( 15.07208474345548055, -141.7963818439230010, 2.500000000000000000 ) ) ;
#22275=CARTESIAN_POINT ( 'NONE',  ( 12.50000000000000000, -132.5000000000000000, -2.500000000000000000 ) ) ;
#22280=FACE_OUTER_BOUND ( 'NONE', #14887, .T. ) ;
#22322=EDGE_LOOP ( 'NONE', ( #67407, #38580, #26981, #25688 ) ) ;
#22329=CARTESIAN_POINT ( 'NONE',  ( 12.13205353604972991, -140.1820037904669789, 5.500000000000000000 ) ) ;
#22335=ADVANCED_FACE ( 'NONE', ( #45180 ), #33132, .F. ) ;
#22369=ORIENTED_EDGE ( 'NONE', *, *, #73650, .T. ) ;
#22389=CARTESIAN_POINT ( 'NONE',  ( -11.59517495878806947, -96.12423995607481686, -5.500000000000000000 ) ) ;
#22393=ORIENTED_EDGE ( 'NONE', *, *, #24199, .T. ) ;
#22424=ORIENTED_EDGE ( 'NONE', *, *, #3341, .F. ) ;
#22436=PLANE ( 'NONE',  #42425 ) ;
#22455=CARTESIAN_POINT ( 'NONE',  ( 70.53423027509757048, -217.0820393249931044, 5.500000000000000000 ) ) ;
#22467=LINE ( 'NONE', #32982, #35275 ) ;
#22501=ORIENTED_EDGE ( 'NONE', *, *, #25204, .T. ) ;
#22504=EDGE_LOOP ( 'NONE', ( #5482, #22117, #8191, #63831 ) ) ;
#22520=AXIS2_PLACEMENT_3D ( 'NONE', #41351, #34223, #6050 ) ;
#22521=CARTESIAN_POINT ( 'NONE',  ( 23.49916127795269460, -121.5130826919798039, 5.500000000000000000 ) ) ;
#22533=EDGE_CURVE ( 'NONE', #9134, #42185, #6441, .T. ) ;
#22551=CARTESIAN_POINT ( 'NONE',  ( -19.90058851926621131, -132.5883508287165853, 5.500000000000000000 ) ) ;
#22562=FACE_OUTER_BOUND ( 'NONE', #9620, .T. ) ;
#22568=EDGE_CURVE ( 'NONE', #40794, #59498, #71045, .T. ) ;
#22577=EDGE_CURVE ( 'NONE', #44562, #54121, #30821, .T. ) ;
#22585=ORIENTED_EDGE ( 'NONE', *, *, #51, .F. ) ;
#22611=EDGE_CURVE ( 'NONE', #16194, #68284, #31565, .T. ) ;
#22629=FACE_OUTER_BOUND ( 'NONE', #26068, .T. ) ;
#22633=LINE ( 'NONE', #14203, #51063 ) ;
#22666=AXIS2_PLACEMENT_3D ( 'NONE', #8377, #2775, #38053 ) ;
#22682=LINE ( 'NONE', #29400, #52850 ) ;
#22691=CARTESIAN_POINT ( 'NONE',  ( -18.24502636017238899, -100.7225776329765665, -2.500000000000000444 ) ) ;
#22707=ORIENTED_EDGE ( 'NONE', *, *, #70119, .T. ) ;
#22734=ORIENTED_EDGE ( 'NONE', *, *, #39381, .T. ) ;
#22742=EDGE_LOOP ( 'NONE', ( #37639, #72388, #22967, #38432 ) ) ;
#22746=ORIENTED_EDGE ( 'NONE', *, *, #15779, .F. ) ;
#22772=EDGE_CURVE ( 'NONE', #40406, #28951, #33804, .T. ) ;
#22797=ADVANCED_FACE ( 'NONE', ( #10493 ), #39454, .F. ) ;
#22807=ORIENTED_EDGE ( 'NONE', *, *, #32557, .T. ) ;
#22812=CARTESIAN_POINT ( 'NONE',  ( -26.29030328629083968, -123.6496510949466341, 5.500000000000000000 ) ) ;
#22818=CARTESIAN_POINT ( 'NONE',  ( 20.85212586905262100, -130.9402397935870965, 5.500000000000000000 ) ) ;
#22830=CARTESIAN_POINT ( 'NONE',  ( -26.29030328629083968, -123.6496510949466341, -5.500000000000000000 ) ) ;
#22841=ORIENTED_EDGE ( 'NONE', *, *, #52210, .F. ) ;
#22856=VERTEX_POINT ( 'NONE', #41297 ) ;
#22881=EDGE_LOOP ( 'NONE', ( #66751, #36245, #27644, #67300 ) ) ;
#22892=ORIENTED_EDGE ( 'NONE', *, *, #53898, .F. ) ;
#22927=CARTESIAN_POINT ( 'NONE',  ( -23.54415474984308787, -120.4156646670583086, -5.500000000000000000 ) ) ;
#22928=LINE ( 'NONE', #50359, #55054 ) ;
#22933=ORIENTED_EDGE ( 'NONE', *, *, #41012, .F. ) ;
#22937=FACE_OUTER_BOUND ( 'NONE', #59821, .T. ) ;
#22947=ORIENTED_EDGE ( 'NONE', *, *, #2113, .T. ) ;
#22948=DIRECTION ( 'NONE',  ( -0.7585478161175716050, -0.6516173805718067369, 0.000000000000000000 ) ) ;
#22967=ORIENTED_EDGE ( 'NONE', *, *, #3191, .F. ) ;
#22969=ORIENTED_EDGE ( 'NONE', *, *, #71813, .T. ) ;
#22990=EDGE_CURVE ( 'NONE', #27599, #13677, #64236, .T. ) ;
#23002=VECTOR ( 'NONE', #2405, 1000.000000000000000 ) ;
#23027=LINE ( 'NONE', #52318, #33249 ) ;
#23031=DIRECTION ( 'NONE',  ( -0.9781476007338069101, 0.2079116908177532363, 0.000000000000000000 ) ) ;
#23060=AXIS2_PLACEMENT_3D ( 'NONE', #2101, #65595, #42659 ) ;
#23082=PLANE ( 'NONE',  #72177 ) ;
#23083=DIRECTION ( 'NONE',  ( 0.1850432970638667407, -0.9827303690289282967, 0.000000000000000000 ) ) ;
#23086=DIRECTION ( 'NONE',  ( -0.000000000000000000, -0.000000000000000000, 1.000000000000000000 ) ) ;
#23095=LINE ( 'NONE', #18178, #56817 ) ;
#23100=PLANE ( 'NONE',  #21817 ) ;
#23112=PLANE ( 'NONE',  #12699 ) ;
#23125=VERTEX_POINT ( 'NONE', #248 ) ;
#23129=ORIENTED_EDGE ( 'NONE', *, *, #53726, .F. ) ;
#23156=CARTESIAN_POINT ( 'NONE',  ( -0.8815729230226008184, -93.47222532549339746, 5.500000000000000000 ) ) ;
#23176=PLANE ( 'NONE',  #66647 ) ;
#23181=LINE ( 'NONE', #11874, #6099 ) ;
#23183=CARTESIAN_POINT ( 'NONE',  ( -21.67772167707813935, -110.8034581014852762, -5.500000000000000000 ) ) ;
#23251=PLANE ( 'NONE',  #8356 ) ;
#23282=LINE ( 'NONE', #63880, #13043 ) ;
#23286=CARTESIAN_POINT ( 'NONE',  ( -23.97194136764370498, -131.3950000906648938, 5.500000000000000000 ) ) ;
#23315=ORIENTED_EDGE ( 'NONE', *, *, #72724, .F. ) ;
#23317=ORIENTED_EDGE ( 'NONE', *, *, #59013, .T. ) ;
#23325=VECTOR ( 'NONE', #38712, 1000.000000000000000 ) ;
#23345=CARTESIAN_POINT ( 'NONE',  ( 12.50000000000000000, -132.5000000000000000, 2.500000000000000000 ) ) ;
#23360=EDGE_CURVE ( 'NONE', #29293, #70940, #45310, .T. ) ;
#23375=DIRECTION ( 'NONE',  ( -0.5687579148473765889, 0.8225049752423776450, 0.000000000000000000 ) ) ;
#23392=DIRECTION ( 'NONE',  ( 0.000000000000000000, 1.000000000000000000, 0.000000000000000000 ) ) ;
#23402=EDGE_CURVE ( 'NONE', #44417, #30226, #62222, .T. ) ;
#23427=DIRECTION ( 'NONE',  ( 0.3311129884571281101, 0.9435911131814402886, -0.000000000000000000 ) ) ;
#23529=AXIS2_PLACEMENT_3D ( 'NONE', #41454, #58371, #29783 ) ;
#23530=VERTEX_POINT ( 'NONE', #13661 ) ;
#23533=FACE_OUTER_BOUND ( 'NONE', #73958, .T. ) ;
#23556=VERTEX_POINT ( 'NONE', #53894 ) ;
#23559=VERTEX_POINT ( 'NONE', #59541 ) ;
#23567=CARTESIAN_POINT ( 'NONE',  ( 0.000000000000000000, -120.0000000000000000, 2.500000000000000000 ) ) ;
#23571=LINE ( 'NONE', #35584, #41781 ) ;
#23575=ORIENTED_EDGE ( 'NONE', *, *, #72485, .T. ) ;
#23591=ORIENTED_EDGE ( 'NONE', *, *, #2011, .F. ) ;
#23620=DIRECTION ( 'NONE',  ( -0.7273375899149802093, 0.6862798483830544471, 0.000000000000000000 ) ) ;
#23623=ORIENTED_EDGE ( 'NONE', *, *, #5102, .F. ) ;
#23629=DIRECTION ( 'NONE',  ( -0.9966891607226785466, -0.08130631524009969413, 0.000000000000000000 ) ) ;
#23641=DIRECTION ( 'NONE',  ( -0.000000000000000000, -0.000000000000000000, -1.000000000000000000 ) ) ;
#23642=VECTOR ( 'NONE', #27239, 1000.000000000000114 ) ;
#23662=EDGE_CURVE ( 'NONE', #42171, #56693, #44090, .T. ) ;
#23667=EDGE_CURVE ( 'NONE', #73780, #11355, #54993, .T. ) ;
#23677=EDGE_LOOP ( 'NONE', ( #8039, #18598, #29548, #70254 ) ) ;
#23683=ORIENTED_EDGE ( 'NONE', *, *, #57213, .T. ) ;
#23686=DIRECTION ( 'NONE',  ( -0.000000000000000000, -0.000000000000000000, -1.000000000000000000 ) ) ;
#23701=ORIENTED_EDGE ( 'NONE', *, *, #57302, .T. ) ;
#23711=CARTESIAN_POINT ( 'NONE',  ( -119.3426274441927433, -132.5434155921188619, 5.500000000000000000 ) ) ;
#23712=CARTESIAN_POINT ( 'NONE',  ( -17.26469406256017791, -140.1601175325492648, 5.500000000000000000 ) ) ;
#23718=DIRECTION ( 'NONE',  ( -0.9918136447140101231, 0.1276937514489694114, 0.000000000000000000 ) ) ;
#23729=VECTOR ( 'NONE', #55196, 1000.000000000000000 ) ;
#23750=ORIENTED_EDGE ( 'NONE', *, *, #5299, .T. ) ;
#23753=ORIENTED_EDGE ( 'NONE', *, *, #10595, .F. ) ;
#23764=CARTESIAN_POINT ( 'NONE',  ( -3.961125083139900749, -143.2122702051246677, 5.500000000000000000 ) ) ;
#23802=ORIENTED_EDGE ( 'NONE', *, *, #65880, .T. ) ;
#23821=( NAMED_UNIT ( * ) SI_UNIT ( $, .STERADIAN. ) SOLID_ANGLE_UNIT ( ) );
#23862=ORIENTED_EDGE ( 'NONE', *, *, #58465, .F. ) ;
#23870=CARTESIAN_POINT ( 'NONE',  ( -22.53294031248082163, -134.0273518838794757, 2.500000000000000000 ) ) ;
#23875=AXIS2_PLACEMENT_3D ( 'NONE', #74119, #73742, #33903 ) ;
#23889=CARTESIAN_POINT ( 'NONE',  ( 24.95699195200416654, -110.9640411295978595, 5.500000000000000000 ) ) ;
#23897=SHAPE_REPRESENTATION ( 'Sliding Dog Clutch Collar', ( #43395 ), #7372 ) ;
#23903=VERTEX_POINT ( 'NONE', #69521 ) ;
#23907=VECTOR ( 'NONE', #13812, 1000.000000000000000 ) ;
#23924=DIRECTION ( 'NONE',  ( 0.000000000000000000, 1.000000000000000000, 0.000000000000000000 ) ) ;
#23992=LINE ( 'NONE', #35995, #37234 ) ;
#23993=CARTESIAN_POINT ( 'NONE',  ( -11.59517495878806947, -96.12423995607481686, -2.500000000000000000 ) ) ;
#24026=CARTESIAN_POINT ( 'NONE',  ( -30.50000000000000000, -120.0000000000000000, 2.500000000000000000 ) ) ;
#24041=EDGE_CURVE ( 'NONE', #105, #54047, #48073, .T. ) ;
#24042=CARTESIAN_POINT ( 'NONE',  ( 20.10151712711562766, -102.7321394148470830, 2.500000000000000000 ) ) ;
#24048=DIRECTION ( 'NONE',  ( -0.9918136447140101231, 0.1276937514489694114, 0.000000000000000000 ) ) ;
#24079=ORIENTED_EDGE ( 'NONE', *, *, #10538, .T. ) ;
#24081=CARTESIAN_POINT ( 'NONE',  ( 6.377742925735834234, -145.7647898336708181, 5.500000000000000000 ) ) ;
#24100=CARTESIAN_POINT ( 'NONE',  ( -12.50000000000000000, -107.5000000000000000, -2.500000000000000000 ) ) ;
#24111=EDGE_CURVE ( 'NONE', #46803, #43453, #56309, .T. ) ;
#24122=AXIS2_PLACEMENT_3D ( 'NONE', #17527, #57022, #40458 ) ;
#24126=ADVANCED_FACE ( 'NONE', ( #10814 ), #68334, .F. ) ;
#24129=PRESENTATION_STYLE_ASSIGNMENT (( #1598 ) ) ;
#24139=VECTOR ( 'NONE', #5137, 1000.000000000000227 ) ;
#24146=PLANE ( 'NONE',  #71218 ) ;
#24151=CARTESIAN_POINT ( 'NONE',  ( -25.50183398199384754, -112.6408924756582053, -5.500000000000000000 ) ) ;
#24181=ORIENTED_EDGE ( 'NONE', *, *, #49690, .F. ) ;
#24199=EDGE_CURVE ( 'NONE', #42171, #61202, #22467, .T. ) ;
#24212=ORIENTED_EDGE ( 'NONE', *, *, #55359, .T. ) ;
#24220=ADVANCED_FACE ( 'NONE', ( #67584 ), #53254, .F. ) ;
#24229=VECTOR ( 'NONE', #13541, 1000.000000000000000 ) ;
#24231=ORIENTED_EDGE ( 'NONE', *, *, #36343, .T. ) ;
#24234=AXIS2_PLACEMENT_3D ( 'NONE', #266, #17870, #41543 ) ;
#24277=EDGE_LOOP ( 'NONE', ( #37302, #70006, #61988, #13746 ) ) ;
#24310=DIRECTION ( 'NONE',  ( -0.9227826878668545785, -0.3853207896976533209, 0.000000000000000000 ) ) ;
#24349=CARTESIAN_POINT ( 'NONE',  ( -0.4301293587032979371, -118.5629931333561871, -2.500000000000000000 ) ) ;
#24364=ORIENTED_EDGE ( 'NONE', *, *, #58896, .F. ) ;
#24392=VECTOR ( 'NONE', #72520, 1000.000000000000114 ) ;
#24399=ORIENTED_EDGE ( 'NONE', *, *, #42515, .T. ) ;
#24406=PLANE ( 'NONE',  #40112 ) ;
#24407=EDGE_LOOP ( 'NONE', ( #63043, #58762, #51993, #50007 ) ) ;
#24412=CARTESIAN_POINT ( 'NONE',  ( 13.83832728059186046, -142.6495187161941089, -2.500000000000000444 ) ) ;
#24423=DIRECTION ( 'NONE',  ( 0.000000000000000000, 0.000000000000000000, 1.000000000000000000 ) ) ;
#24434=VERTEX_POINT ( 'NONE', #2160 ) ;
#24444=LINE ( 'NONE', #65779, #51265 ) ;
#24488=VERTEX_POINT ( 'NONE', #49456 ) ;
#24501=CARTESIAN_POINT ( 'NONE',  ( -7.670864526094549163, -97.73662565058241114, 5.500000000000000000 ) ) ;
#24548=CARTESIAN_POINT ( 'NONE',  ( 0.000000000000000000, -120.0000000000000000, 2.500000000000000000 ) ) ;
#24549=AXIS2_PLACEMENT_3D ( 'NONE', #2427, #54620, #9120 ) ;
#24604=CARTESIAN_POINT ( 'NONE',  ( -23.30023580412278505, -123.4057321492263384, -5.500000000000000000 ) ) ;
#24610=CARTESIAN_POINT ( 'NONE',  ( 26.47460221209471598, -121.8961639463267090, 5.500000000000000000 ) ) ;
#24624=FACE_OUTER_BOUND ( 'NONE', #61074, .T. ) ;
#24630=EDGE_CURVE ( 'NONE', #40375, #22856, #41063, .T. ) ;
#24647=PLANE ( 'NONE',  #33718 ) ;
#24649=CARTESIAN_POINT ( 'NONE',  ( -1.233757462863590115, -120.8531368722710795, -2.500000000000000000 ) ) ;
#24671=ORIENTED_EDGE ( 'NONE', *, *, #40087, .F. ) ;
#24707=DIRECTION ( 'NONE',  ( 0.000000000000000000, -1.000000000000000000, 0.000000000000000000 ) ) ;
#24721=VECTOR ( 'NONE', #1296, 1000.000000000000114 ) ;
#24763=LINE ( 'NONE', #24042, #32966 ) ;
#24771=ORIENTED_EDGE ( 'NONE', *, *, #23667, .T. ) ;
#24783=ORIENTED_EDGE ( 'NONE', *, *, #5102, .T. ) ;
#24792=FACE_OUTER_BOUND ( 'NONE', #13876, .T. ) ;
#24801=ORIENTED_EDGE ( 'NONE', *, *, #60554, .T. ) ;
#24830=CARTESIAN_POINT ( 'NONE',  ( -17.26469406256017791, -140.1601175325492648, 2.500000000000000000 ) ) ;
#24858=FACE_BOUND ( 'NONE', #51780, .T. ) ;
#24914=DIRECTION ( 'NONE',  ( -0.9966891607226785466, -0.08130631524010122069, 0.000000000000000000 ) ) ;
#24916=AXIS2_PLACEMENT_3D ( 'NONE', #70941, #65694, #64577 ) ;
#24926=SHAPE_REPRESENTATION_RELATIONSHIP ( 'NONE' , 'NONE' ,  #23897, #28332 ) ;
#24951=ORIENTED_EDGE ( 'NONE', *, *, #55359, .F. ) ;
#24968=ADVANCED_FACE ( 'NONE', ( #74055 ), #11636, .F. ) ;
#24990=ORIENTED_EDGE ( 'NONE', *, *, #52280, .F. ) ;
#24993=VERTEX_POINT ( 'NONE', #69538 ) ;
#25000=CARTESIAN_POINT ( 'NONE',  ( -35.50000000000000711, -120.0000000000000000, 2.500000000000000000 ) ) ;
#25006=LINE ( 'NONE', #1754, #29439 ) ;
#25023=EDGE_CURVE ( 'NONE', #11010, #33943, #38919, .T. ) ;
#25037=DIRECTION ( 'NONE',  ( -0.9227826878668540234, -0.3853207896976547642, 0.000000000000000000 ) ) ;
#25061=CARTESIAN_POINT ( 'NONE',  ( -17.26469406256017791, -140.1601175325492648, -5.500000000000000000 ) ) ;
#25078=CARTESIAN_POINT ( 'NONE',  ( -114.1267819554185365, -82.91796067500661138, -5.500000000000000000 ) ) ;
#25115=DIRECTION ( 'NONE',  ( 0.9918136447140100120, -0.1276937514489704939, 0.000000000000000000 ) ) ;
#25119=DIRECTION ( 'NONE',  ( 0.8541291221503275466, -0.5200609990132993854, 0.000000000000000000 ) ) ;
#25120=ADVANCED_FACE ( 'NONE', ( #1160 ), #58256, .F. ) ;
#25148=ORIENTED_EDGE ( 'NONE', *, *, #7664, .T. ) ;
#25150=CARTESIAN_POINT ( 'NONE',  ( -25.00516449930816876, -111.2255058058861010, -2.500000000000000000 ) ) ;
#25171=CARTESIAN_POINT ( 'NONE',  ( -89.17737905728745318, -39.70432723693717492, -5.500000000000000000 ) ) ;
#25173=ORIENTED_EDGE ( 'NONE', *, *, #18379, .T. ) ;
#25181=EDGE_LOOP ( 'NONE', ( #58811, #32714, #22841, #63309 ) ) ;
#25196=ADVANCED_FACE ( 'NONE', ( #13851 ), #20621, .F. ) ;
#25198=CARTESIAN_POINT ( 'NONE',  ( 5.822613034544236399, -142.8165987265839760, 5.500000000000000000 ) ) ;
#25203=DIRECTION ( 'NONE',  ( -0.9827303690289279636, -0.1850432970638682117, 0.000000000000000000 ) ) ;
#25204=EDGE_CURVE ( 'NONE', #59498, #17376, #15337, .T. ) ;
#25222=ADVANCED_FACE ( 'NONE', ( #66128 ), #71361, .F. ) ;
#25262=CARTESIAN_POINT ( 'NONE',  ( -20.30386590532152979, -102.9045904027214959, 5.500000000000000000 ) ) ;
#25278=CARTESIAN_POINT ( 'NONE',  ( -23.54415474984308787, -120.4156646670583086, 5.500000000000000000 ) ) ;
#25288=FACE_OUTER_BOUND ( 'NONE', #1184, .T. ) ;
#25303=FACE_BOUND ( 'NONE', #14566, .T. ) ;
#25304=CARTESIAN_POINT ( 'NONE',  ( 3.429551818649054340, -146.3199197248623875, -2.500000000000000444 ) ) ;
#25318=VECTOR ( 'NONE', #35532, 1000.000000000000000 ) ;
#25337=ORIENTED_EDGE ( 'NONE', *, *, #4705, .F. ) ;
#25348=DIRECTION ( 'NONE',  ( -0.9580045777625456616, -0.2867529058022021404, 0.000000000000000000 ) ) ;
#25366=FACE_OUTER_BOUND ( 'NONE', #28378, .T. ) ;
#25381=DIRECTION ( 'NONE',  ( 0.1276937514489679681, 0.9918136447140103451, 0.000000000000000000 ) ) ;
#25391=CARTESIAN_POINT ( 'NONE',  ( -7.572224309238338336, -145.4393675041377492, -5.500000000000000000 ) ) ;
#25410=ORIENTED_EDGE ( 'NONE', *, *, #18307, .F. ) ;
#25430=ORIENTED_EDGE ( 'NONE', *, *, #53726, .T. ) ;
#25463=DIRECTION ( 'NONE',  ( 0.9435911131814398445, -0.3311129884571295534, 0.000000000000000000 ) ) ;
#25486=CARTESIAN_POINT ( 'NONE',  ( -15.44521549751111422, -137.7748507232956001, -5.500000000000000000 ) ) ;
#25489=VERTEX_POINT ( 'NONE', #58167 ) ;
#25531=ORIENTED_EDGE ( 'NONE', *, *, #32943, .F. ) ;
#25555=CARTESIAN_POINT ( 'NONE',  ( 35.50000000000000711, -120.0000000000000000, 2.500000000000000000 ) ) ;
#25570=EDGE_CURVE ( 'NONE', #6148, #50088, #17945, .T. ) ;
#25599=CARTESIAN_POINT ( 'NONE',  ( -23.97194136764370498, -131.3950000906648938, 5.500000000000000000 ) ) ;
#25624=EDGE_LOOP ( 'NONE', ( #37453, #40106, #43574, #57244 ) ) ;
#25638=CARTESIAN_POINT ( 'NONE',  ( -19.90058851926621131, -132.5883508287165853, 5.500000000000000000 ) ) ;
#25650=EDGE_CURVE ( 'NONE', #973, #64962, #19414, .T. ) ;
#25655=CARTESIAN_POINT ( 'NONE',  ( -13.05994868825747446, -139.5943292883446532, -5.500000000000000000 ) ) ;
#25683=ADVANCED_FACE ( 'NONE', ( #7773 ), #20900, .T. ) ;
#25685=LINE ( 'NONE', #71904, #7874 ) ;
#25688=ORIENTED_EDGE ( 'NONE', *, *, #22533, .T. ) ;
#25695=VERTEX_POINT ( 'NONE', #25061 ) ;
#25805=LINE ( 'NONE', #20544, #14623 ) ;
#25809=ORIENTED_EDGE ( 'NONE', *, *, #41926, .T. ) ;
#25811=EDGE_CURVE ( 'NONE', #63004, #55103, #67510, .T. ) ;
#25816=DIRECTION ( 'NONE',  ( -0.000000000000000000, -0.000000000000000000, 1.000000000000000000 ) ) ;
#25825=EDGE_CURVE ( 'NONE', #1781, #17454, #61879, .T. ) ;
#25829=VECTOR ( 'NONE', #29185, 1000.000000000000000 ) ;
#25854=LINE ( 'NONE', #71708, #69109 ) ;
#25866=DIRECTION ( 'NONE',  ( 0.3853207896976523772, -0.9227826878668550226, 0.000000000000000000 ) ) ;
#25869=EDGE_LOOP ( 'NONE', ( #2845, #27163, #49557, #14885 ) ) ;
#25870=VECTOR ( 'NONE', #45350, 1000.000000000000000 ) ;
#25883=ORIENTED_EDGE ( 'NONE', *, *, #1253, .T. ) ;
#25906=ORIENTED_EDGE ( 'NONE', *, *, #48196, .T. ) ;
#25908=DIRECTION ( 'NONE',  ( -0.5200609990132993854, -0.8541291221503275466, 0.000000000000000000 ) ) ;
#25932=VECTOR ( 'NONE', #45996, 1000.000000000000114 ) ;
#25937=CARTESIAN_POINT ( 'NONE',  ( -23.25244084006223133, -132.7111759872722416, 2.500000000000000000 ) ) ;
#25946=ORIENTED_EDGE ( 'NONE', *, *, #50756, .F. ) ;
#25948=CARTESIAN_POINT ( 'NONE',  ( 14.59956846177685996, -138.4757300459248484, 5.500000000000000000 ) ) ;
#25995=DIRECTION ( 'NONE',  ( 0.8774505977381978905, 0.4796670183876304283, -0.000000000000000000 ) ) ;
#26001=FACE_OUTER_BOUND ( 'NONE', #54630, .T. ) ;
#26020=VERTEX_POINT ( 'NONE', #51703 ) ;
#26036=DIRECTION ( 'NONE',  ( 0.02332147558787822997, 0.9997280174009349762, 0.000000000000000000 ) ) ;
#26049=VERTEX_POINT ( 'NONE', #26453 ) ;
#26062=EDGE_CURVE ( 'NONE', #68933, #54089, #37386, .T. ) ;
#26067=DIRECTION ( 'NONE',  ( -0.000000000000000000, -0.000000000000000000, -1.000000000000000000 ) ) ;
#26068=EDGE_LOOP ( 'NONE', ( #49362, #41417, #8184, #67520 ) ) ;
#26079=CARTESIAN_POINT ( 'NONE',  ( 8.700667342345820288, -98.11853780484867116, 5.500000000000000000 ) ) ;
#26114=CARTESIAN_POINT ( 'NONE',  ( 14.59956846177685996, -138.4757300459248484, 5.500000000000000000 ) ) ;
#26116=LINE ( 'NONE', #26496, #43088 ) ;
#26126=FACE_OUTER_BOUND ( 'NONE', #35617, .T. ) ;
#26148=CARTESIAN_POINT ( 'NONE',  ( -16.06301359042743115, -102.7814171781257357, 5.500000000000000000 ) ) ;
#26154=VERTEX_POINT ( 'NONE', #20064 ) ;
#26157=AXIS2_PLACEMENT_3D ( 'NONE', #58519, #63443, #35221 ) ;
#26197=VECTOR ( 'NONE', #65892, 1000.000000000000000 ) ;
#26215=CARTESIAN_POINT ( 'NONE',  ( -15.44521549751111422, -137.7748507232956001, 2.500000000000000000 ) ) ;
#26217=VECTOR ( 'NONE', #40066, 1000.000000000000114 ) ;
#26246=AXIS2_PLACEMENT_3D ( 'NONE', #25948, #8289, #19562 ) ;
#26296=AXIS2_PLACEMENT_3D ( 'NONE', #7603, #30516, #69645 ) ;
#26330=CARTESIAN_POINT ( 'NONE',  ( 1.233757462863572574, -119.1468631277289347, -2.500000000000000000 ) ) ;
#26339=CARTESIAN_POINT ( 'NONE',  ( -0.8815729230226008184, -93.47222532549339746, -5.500000000000000000 ) ) ;
#26348=VERTEX_POINT ( 'NONE', #58357 ) ;
#26372=DIRECTION ( 'NONE',  ( 0.3311129884571304971, 0.9435911131814395114, -0.000000000000000000 ) ) ;
#26387=EDGE_CURVE ( 'NONE', #70060, #28874, #59603, .T. ) ;
#26399=CARTESIAN_POINT ( 'NONE',  ( -32.50000000000000000, -120.0000000000000000, 2.500000000000000000 ) ) ;
#26402=LINE ( 'NONE', #45193, #31734 ) ;
#26453=CARTESIAN_POINT ( 'NONE',  ( 21.85433023846371370, -135.0628101570779620, -5.500000000000000000 ) ) ;
#26494=DIRECTION ( 'NONE',  ( -0.1276937514489679404, -0.9918136447140103451, 0.000000000000000000 ) ) ;
#26496=CARTESIAN_POINT ( 'NONE',  ( 19.12409105625795291, -101.5943176906707919, 5.500000000000000000 ) ) ;
#26554=LINE ( 'NONE', #50216, #59447 ) ;
#26555=DIRECTION ( 'NONE',  ( -0.2867529058022021404, 0.9580045777625456616, 0.000000000000000000 ) ) ;
#26559=ORIENTED_EDGE ( 'NONE', *, *, #22568, .T. ) ;
#26574=CARTESIAN_POINT ( 'NONE',  ( -12.50000000000000000, -132.5000000000000000, 2.500000000000000000 ) ) ;
#26575=VECTOR ( 'NONE', #36196, 1000.000000000000000 ) ;
#26581=LINE ( 'NONE', #3684, #38801 ) ;
#26604=CARTESIAN_POINT ( 'NONE',  ( -24.50849501662245800, -109.8101191361138831, -5.500000000000000000 ) ) ;
#26626=LINE ( 'NONE', #38286, #65902 ) ;
#26637=DIRECTION ( 'NONE',  ( 0.1276937514489694392, 0.9918136447140102341, -0.000000000000000000 ) ) ;
#26653=LINE ( 'NONE', #33032, #54275 ) ;
#26662=DIRECTION ( 'NONE',  ( -0.9038112904824846527, 0.4279312458752990711, 0.000000000000000000 ) ) ;
#26672=CARTESIAN_POINT ( 'NONE',  ( 2.117611129180199558, -93.54218975225703048, 5.500000000000000000 ) ) ;
#26690=ORIENTED_EDGE ( 'NONE', *, *, #29854, .T. ) ;
#26709=ORIENTED_EDGE ( 'NONE', *, *, #73298, .F. ) ;
#26717=LINE ( 'NONE', #10178, #9028 ) ;
#26722=PLANE ( 'NONE',  #73279 ) ;
#26734=CARTESIAN_POINT ( 'NONE',  ( -25.50183398199384754, -112.6408924756582053, 5.500000000000000000 ) ) ;
#26760=DIRECTION ( 'NONE',  ( 0.1850432970638656582, -0.9827303690289285187, 0.000000000000000000 ) ) ;
#26779=VECTOR ( 'NONE', #60020, 1000.000000000000227 ) ;
#26782=VECTOR ( 'NONE', #15116, 1000.000000000000000 ) ;
#26806=ORIENTED_EDGE ( 'NONE', *, *, #58220, .F. ) ;
#26807=ORIENTED_EDGE ( 'NONE', *, *, #58896, .T. ) ;
#26832=DIRECTION ( 'NONE',  ( -0.1045284632676570929, 0.9945218953682730678, 0.000000000000000000 ) ) ;
#26838=EDGE_CURVE ( 'NONE', #71076, #23556, #64995, .T. ) ;
#26858=LINE ( 'NONE', #72702, #60524 ) ;
#26861=DIRECTION ( 'NONE',  ( -0.000000000000000000, -0.000000000000000000, -1.000000000000000000 ) ) ;
#26875=VERTEX_POINT ( 'NONE', #14864 ) ;
#26937=CYLINDRICAL_SURFACE ( 'NONE', #45117, 30.50000000000000000 ) ;
#26938=VECTOR ( 'NONE', #60124, 1000.000000000000114 ) ;
#26950=CARTESIAN_POINT ( 'NONE',  ( -18.24502636017238899, -100.7225776329765665, 5.500000000000000000 ) ) ;
#26957=FACE_OUTER_BOUND ( 'NONE', #42723, .T. ) ;
#26958=VECTOR ( 'NONE', #62804, 1000.000000000000114 ) ;
#26981=ORIENTED_EDGE ( 'NONE', *, *, #42204, .T. ) ;
#26990=ORIENTED_EDGE ( 'NONE', *, *, #19522, .T. ) ;
#26994=DIRECTION ( 'NONE',  ( -0.000000000000000000, -0.000000000000000000, -1.000000000000000000 ) ) ;
#27004=CARTESIAN_POINT ( 'NONE',  ( 2.047646702416564768, -96.54137380445985173, 5.500000000000000000 ) ) ;
#27007=VERTEX_POINT ( 'NONE', #68560 ) ;
#27040=EDGE_CURVE ( 'NONE', #49118, #37730, #39983, .T. ) ;
#27067=ORIENTED_EDGE ( 'NONE', *, *, #35635, .T. ) ;
#27074=LINE ( 'NONE', #20707, #29624 ) ;
#27083=ORIENTED_EDGE ( 'NONE', *, *, #25825, .T. ) ;
#27087=VERTEX_POINT ( 'NONE', #19988 ) ;
#27089=ORIENTED_EDGE ( 'NONE', *, *, #656, .T. ) ;
#27090=CARTESIAN_POINT ( 'NONE',  ( 2.047646702416564768, -96.54137380445985173, 2.500000000000000000 ) ) ;
#27093=ORIENTED_EDGE ( 'NONE', *, *, #50560, .F. ) ;
#27101=CARTESIAN_POINT ( 'NONE',  ( 12.50000000000000000, -132.5000000000000000, 2.500000000000000000 ) ) ;
#27111=AXIS2_PLACEMENT_3D ( 'NONE', #33228, #16323, #21203 ) ;
#27149=ORIENTED_EDGE ( 'NONE', *, *, #49690, .T. ) ;
#27158=ORIENTED_EDGE ( 'NONE', *, *, #22611, .F. ) ;
#27163=ORIENTED_EDGE ( 'NONE', *, *, #37337, .F. ) ;
#27168=ORIENTED_EDGE ( 'NONE', *, *, #73476, .F. ) ;
#27200=DIRECTION ( 'NONE',  ( -0.000000000000000000, -0.000000000000000000, -1.000000000000000000 ) ) ;
#27225=PLANE ( 'NONE',  #31370 ) ;
#27238=ORIENTED_EDGE ( 'NONE', *, *, #17510, .T. ) ;
#27239=DIRECTION ( 'NONE',  ( -0.9827303690289279636, -0.1850432970638682117, 0.000000000000000000 ) ) ;
#27245=ORIENTED_EDGE ( 'NONE', *, *, #4042, .F. ) ;
#27249=EDGE_CURVE ( 'NONE', #61202, #44676, #44423, .T. ) ;
#27286=ORIENTED_EDGE ( 'NONE', *, *, #26387, .F. ) ;
#27290=ORIENTED_EDGE ( 'NONE', *, *, #31759, .T. ) ;
#27302=DIRECTION ( 'NONE',  ( 0.9135454576426059736, -0.4067366430757887730, 0.000000000000000000 ) ) ;
#27369=LINE ( 'NONE', #40155, #54984 ) ;
#27384=ORIENTED_EDGE ( 'NONE', *, *, #61277, .T. ) ;
#27400=CARTESIAN_POINT ( 'NONE',  ( -8.826826895187510402, -94.96827758698185562, 5.500000000000000000 ) ) ;
#27402=AXIS2_PLACEMENT_3D ( 'NONE', #4635, #72641, #4260 ) ;
#27445=CARTESIAN_POINT ( 'NONE',  ( 119.3426274441929280, -132.5434155921172419, -5.500000000000000000 ) ) ;
#27450=EDGE_LOOP ( 'NONE', ( #65464, #67125, #55278, #53565 ) ) ;
#27471=EDGE_CURVE ( 'NONE', #55116, #13677, #45549, .T. ) ;
#27533=DIRECTION ( 'NONE',  ( 0.7273375899149802093, -0.6862798483830544471, 0.000000000000000000 ) ) ;
#27545=EDGE_LOOP ( 'NONE', ( #3149, #10353, #8491, #55655 ) ) ;
#27599=VERTEX_POINT ( 'NONE', #53026 ) ;
#27613=LINE ( 'NONE', #208, #11051 ) ;
#27626=VERTEX_POINT ( 'NONE', #47741 ) ;
#27637=ORIENTED_EDGE ( 'NONE', *, *, #3615, .F. ) ;
#27644=ORIENTED_EDGE ( 'NONE', *, *, #6967, .F. ) ;
#27688=CARTESIAN_POINT ( 'NONE',  ( -10.43921258969510824, -98.89258801967538659, -2.500000000000000000 ) ) ;
#27705=DIRECTION ( 'NONE',  ( -0.8090169943749504489, 0.5877852522924689183, 0.000000000000000000 ) ) ;
#27707=ORIENTED_EDGE ( 'NONE', *, *, #14094, .T. ) ;
#27715=CARTESIAN_POINT ( 'NONE',  ( 35.50000000000000711, -120.0000000000000000, 2.500000000000000000 ) ) ;
#27734=ADVANCED_FACE ( 'NONE', ( #9742 ), #43605, .F. ) ;
#27738=DIRECTION ( 'NONE',  ( -0.5687579148473765889, 0.8225049752423776450, 0.000000000000000000 ) ) ;
#27748=ORIENTED_EDGE ( 'NONE', *, *, #36054, .T. ) ;
#27751=CARTESIAN_POINT ( 'NONE',  ( 12.50000000000000000, -107.5000000000000000, -2.500000000000000000 ) ) ;
#27761=VERTEX_POINT ( 'NONE', #10111 ) ;
#27763=VECTOR ( 'NONE', #54054, 1000.000000000000000 ) ;
#27776=LINE ( 'NONE', #55230, #34462 ) ;
#27782=VECTOR ( 'NONE', #56547, 1000.000000000000114 ) ;
#27803=DIRECTION ( 'NONE',  ( -0.000000000000000000, -0.000000000000000000, -1.000000000000000000 ) ) ;
#27811=FACE_OUTER_BOUND ( 'NONE', #57958, .T. ) ;
#27833=VERTEX_POINT ( 'NONE', #28142 ) ;
#27873=CARTESIAN_POINT ( 'NONE',  ( -22.67106064244953245, -113.6342314410295842, 5.500000000000000000 ) ) ;
#27876=LINE ( 'NONE', #50800, #50958 ) ;
#27951=CARTESIAN_POINT ( 'NONE',  ( 0.1915406271734537980, -118.5122795329289858, -2.500000000000000000 ) ) ;
#27963=ORIENTED_EDGE ( 'NONE', *, *, #53898, .T. ) ;
#27966=DIRECTION ( 'NONE',  ( 0.000000000000000000, 0.000000000000000000, 1.000000000000000000 ) ) ;
#27968=CARTESIAN_POINT ( 'NONE',  ( -12.50000000000000000, -132.5000000000000000, 2.500000000000000000 ) ) ;
#27983=VECTOR ( 'NONE', #10120, 1000.000000000000000 ) ;
#27989=LINE ( 'NONE', #63710, #32280 ) ;
#28024=ORIENTED_EDGE ( 'NONE', *, *, #42132, .F. ) ;
#28047=CARTESIAN_POINT ( 'NONE',  ( 26.09152095774781799, -124.8716048804687375, 5.500000000000000000 ) ) ;
#28063=AXIS2_PLACEMENT_3D ( 'NONE', #7229, #8703, #31620 ) ;
#28064=DIRECTION ( 'NONE',  ( -0.3853207896976523772, 0.9227826878668550226, 0.000000000000000000 ) ) ;
#28065=CARTESIAN_POINT ( 'NONE',  ( 25.81725066941077884, -113.8380548628854854, 2.500000000000000000 ) ) ;
#28082=FACE_OUTER_BOUND ( 'NONE', #52021, .T. ) ;
#28103=FACE_OUTER_BOUND ( 'NONE', #28798, .T. ) ;
#28142=CARTESIAN_POINT ( 'NONE',  ( 23.41451323550360186, -132.5004227906269989, 5.500000000000000000 ) ) ;
#28189=ORIENTED_EDGE ( 'NONE', *, *, #26838, .T. ) ;
#28203=EDGE_CURVE ( 'NONE', #37554, #973, #55426, .T. ) ;
#28204=ORIENTED_EDGE ( 'NONE', *, *, #39675, .T. ) ;
#28209=ORIENTED_EDGE ( 'NONE', *, *, #53883, .F. ) ;
#28230=VECTOR ( 'NONE', #39694, 1000.000000000000114 ) ;
#28277=ORIENTED_EDGE ( 'NONE', *, *, #36405, .F. ) ;
#28280=EDGE_LOOP ( 'NONE', ( #51411, #53950, #5424, #73049 ) ) ;
#28294=CARTESIAN_POINT ( 'NONE',  ( 23.49916127795269105, -121.5130826919798039, -2.500000000000000000 ) ) ;
#28322=LINE ( 'NONE', #21951, #61973 ) ;
#28330=EDGE_CURVE ( 'NONE', #18041, #15423, #74196, .T. ) ;
#28332=ADVANCED_BREP_SHAPE_REPRESENTATION ( '', ( #37782, #43395 ), #7372 ) ;
#28347=VERTEX_POINT ( 'NONE', #35454 ) ;
#28368=VECTOR ( 'NONE', #14676, 1000.000000000000000 ) ;
#28375=CARTESIAN_POINT ( 'NONE',  ( -3.961125083139900749, -143.2122702051246677, 5.500000000000000000 ) ) ;
#28378=EDGE_LOOP ( 'NONE', ( #57201, #69827, #37810, #66663 ) ) ;
#28382=DIRECTION ( 'NONE',  ( 0.6064928550163531940, 0.7950889364178782559, 0.000000000000000000 ) ) ;
#28385=CARTESIAN_POINT ( 'NONE',  ( 26.47460221209471598, -121.8961639463267090, 5.500000000000000000 ) ) ;
#28390=ORIENTED_EDGE ( 'NONE', *, *, #5299, .F. ) ;
#28408=VERTEX_POINT ( 'NONE', #13625 ) ;
#28414=EDGE_CURVE ( 'NONE', #2800, #64355, #59883, .T. ) ;
#28419=PLANE ( 'NONE',  #40148 ) ;
#28423=EDGE_CURVE ( 'NONE', #38008, #46993, #42224, .T. ) ;
#28468=ORIENTED_EDGE ( 'NONE', *, *, #18815, .F. ) ;
#28493=ORIENTED_EDGE ( 'NONE', *, *, #17389, .F. ) ;
#28496=EDGE_CURVE ( 'NONE', #38411, #12079, #64781, .T. ) ;
#28500=EDGE_LOOP ( 'NONE', ( #15428, #33031, #20691, #8917 ) ) ;
#28518=DIRECTION ( 'NONE',  ( -0.000000000000000000, -0.000000000000000000, 1.000000000000000000 ) ) ;
#28521=CARTESIAN_POINT ( 'NONE',  ( -23.97194136764370498, -131.3950000906648938, -5.500000000000000000 ) ) ;
#28522=CARTESIAN_POINT ( 'NONE',  ( 0.7800914985199594032, -118.7188063167744900, -2.500000000000000000 ) ) ;
#28535=EDGE_LOOP ( 'NONE', ( #26709, #23575, #33094, #44295 ) ) ;
#28543=DIRECTION ( 'NONE',  ( -0.000000000000000000, -0.000000000000000000, -1.000000000000000000 ) ) ;
#28556=LINE ( 'NONE', #51499, #59265 ) ;
#28557=EDGE_LOOP ( 'NONE', ( #13844, #5967, #73846, #33747 ) ) ;
#28599=PLANE ( 'NONE',  #6111 ) ;
#28608=EDGE_CURVE ( 'NONE', #52621, #29721, #9467, .T. ) ;
#28625=PLANE ( 'NONE',  #69409 ) ;
#28631=CARTESIAN_POINT ( 'NONE',  ( 12.50000000000000000, -107.5000000000000000, 2.500000000000000000 ) ) ;
#28643=ORIENTED_EDGE ( 'NONE', *, *, #26062, .F. ) ;
#28656=VECTOR ( 'NONE', #12159, 1000.000000000000114 ) ;
#28658=VECTOR ( 'NONE', #59421, 1000.000000000000114 ) ;
#28687=CARTESIAN_POINT ( 'NONE',  ( 30.50000000000000000, -120.0000000000000000, -5.500000000000000000 ) ) ;
#28734=ORIENTED_EDGE ( 'NONE', *, *, #30825, .T. ) ;
#28757=CARTESIAN_POINT ( 'NONE',  ( -4.653126046682595884, -146.1313684676804314, 2.500000000000000000 ) ) ;
#28780=CIRCLE ( 'NONE', #31187, 30.50000000000000000 ) ;
#28798=EDGE_LOOP ( 'NONE', ( #23750, #32535, #1537, #36809 ) ) ;
#28822=LINE ( 'NONE', #50262, #67464 ) ;
#28838=CARTESIAN_POINT ( 'NONE',  ( -21.67772167707813935, -110.8034581014852762, 2.500000000000000000 ) ) ;
#28861=CARTESIAN_POINT ( 'NONE',  ( -23.30023580412278505, -123.4057321492263384, 5.500000000000000000 ) ) ;
#28874=VERTEX_POINT ( 'NONE', #36839 ) ;
#28876=VECTOR ( 'NONE', #42053, 1000.000000000000114 ) ;
#28907=LINE ( 'NONE', #45480, #1784 ) ;
#28941=VERTEX_POINT ( 'NONE', #13171 ) ;
#28944=ORIENTED_EDGE ( 'NONE', *, *, #883, .T. ) ;
#28951=VERTEX_POINT ( 'NONE', #59050 ) ;
#28979=LINE ( 'NONE', #51911, #42334 ) ;
#28986=VECTOR ( 'NONE', #46729, 1000.000000000000114 ) ;
#28991=CARTESIAN_POINT ( 'NONE',  ( -22.67106064244953245, -113.6342314410295842, -5.500000000000000000 ) ) ;
#28997=PLANE ( 'NONE',  #65909 ) ;
#29000=CARTESIAN_POINT ( 'NONE',  ( 16.84844760790522855, -103.5491698323862124, 2.500000000000000000 ) ) ;
#29007=VERTEX_POINT ( 'NONE', #43616 ) ;
#29051=ORIENTED_EDGE ( 'NONE', *, *, #22094, .F. ) ;
#29058=PLANE ( 'NONE',  #23529 ) ;
#29106=VECTOR ( 'NONE', #19178, 1000.000000000000000 ) ;
#29108=ORIENTED_EDGE ( 'NONE', *, *, #19501, .T. ) ;
#29118=ORIENTED_EDGE ( 'NONE', *, *, #38810, .F. ) ;
#29140=FACE_OUTER_BOUND ( 'NONE', #44290, .T. ) ;
#29149=VECTOR ( 'NONE', #52035, 1000.000000000000000 ) ;
#29152=CARTESIAN_POINT ( 'NONE',  ( -0.8815729230226008184, -93.47222532549339746, 5.500000000000000000 ) ) ;
#29160=CYLINDRICAL_SURFACE ( 'NONE', #33504, 30.50000000000000000 ) ;
#29164=CARTESIAN_POINT ( 'NONE',  ( 26.09152095774781444, -124.8716048804687375, 2.500000000000000000 ) ) ;
#29170=CARTESIAN_POINT ( 'NONE',  ( -22.67106064244953245, -113.6342314410295842, 5.500000000000000000 ) ) ;
#29185=DIRECTION ( 'NONE',  ( -0.000000000000000000, -0.000000000000000000, 1.000000000000000000 ) ) ;
#29194=DIRECTION ( 'NONE',  ( 0.9827303690289282967, 0.1850432970638667407, -0.000000000000000000 ) ) ;
#29223=ORIENTED_EDGE ( 'NONE', *, *, #16716, .T. ) ;
#29248=AXIS2_PLACEMENT_3D ( 'NONE', #21327, #38265, #10433 ) ;
#29254=CARTESIAN_POINT ( 'NONE',  ( 0.000000000000000000, -120.0000000000000000, -5.500000000000000000 ) ) ;
#29259=VECTOR ( 'NONE', #41133, 1000.000000000000000 ) ;
#29264=VECTOR ( 'NONE', #42399, 1000.000000000000114 ) ;
#29270=CARTESIAN_POINT ( 'NONE',  ( 16.30584220631899228, -140.9432449716519784, 5.500000000000000000 ) ) ;
#29282=EDGE_CURVE ( 'NONE', #40323, #38913, #1487, .T. ) ;
#29291=CARTESIAN_POINT ( 'NONE',  ( 23.11608002360578240, -124.4885236261218182, 5.500000000000000000 ) ) ;
#29293=VERTEX_POINT ( 'NONE', #2597 ) ;
#29319=LINE ( 'NONE', #47370, #1380 ) ;
#29332=EDGE_CURVE ( 'NONE', #64355, #64095, #19824, .T. ) ;
#29352=CARTESIAN_POINT ( 'NONE',  ( -10.43921258969510824, -98.89258801967538659, 2.500000000000000000 ) ) ;
#29375=EDGE_CURVE ( 'NONE', #38563, #8717, #36377, .T. ) ;
#29389=EDGE_LOOP ( 'NONE', ( #53344, #50012, #29654, #51942 ) ) ;
#29400=CARTESIAN_POINT ( 'NONE',  ( 0.4966694826857007139, -118.5846133302278247, 2.500000000000000000 ) ) ;
#29410=DIRECTION ( 'NONE',  ( -0.9227826878668540234, -0.3853207896976546531, 0.000000000000000000 ) ) ;
#29422=CIRCLE ( 'NONE', #48652, 30.50000000000000000 ) ;
#29430=DIRECTION ( 'NONE',  ( -0.000000000000000000, -0.000000000000000000, -1.000000000000000000 ) ) ;
#29438=DIRECTION ( 'NONE',  ( 1.000000000000000000, 0.000000000000000000, 0.000000000000000000 ) ) ;
#29439=VECTOR ( 'NONE', #41940, 1000.000000000000114 ) ;
#29473=AXIS2_PLACEMENT_3D ( 'NONE', #67347, #15848, #39905 ) ;
#29492=LINE ( 'NONE', #35151, #69255 ) ;
#29505=EDGE_CURVE ( 'NONE', #37728, #49062, #72074, .T. ) ;
#29509=DIRECTION ( 'NONE',  ( -0.1276937514489705217, -0.9918136447140101231, 0.000000000000000000 ) ) ;
#29513=ORIENTED_EDGE ( 'NONE', *, *, #53161, .T. ) ;
#29524=DIRECTION ( 'NONE',  ( -0.000000000000000000, -0.000000000000000000, 1.000000000000000000 ) ) ;
#29526=CARTESIAN_POINT ( 'NONE',  ( 25.81725066941077529, -113.8380548628854854, -5.500000000000000000 ) ) ;
#29537=EDGE_CURVE ( 'NONE', #7680, #31960, #49876, .T. ) ;
#29542=LINE ( 'NONE', #53234, #10000 ) ;
#29548=ORIENTED_EDGE ( 'NONE', *, *, #3103, .F. ) ;
#29576=ORIENTED_EDGE ( 'NONE', *, *, #5800, .F. ) ;
#29584=DIRECTION ( 'NONE',  ( 0.000000000000000000, 0.000000000000000000, 1.000000000000000000 ) ) ;
#29608=LINE ( 'NONE', #46194, #10391 ) ;
#29613=LINE ( 'NONE', #739, #38826 ) ;
#29624=VECTOR ( 'NONE', #15430, 1000.000000000000000 ) ;
#29643=ORIENTED_EDGE ( 'NONE', *, *, #58465, .T. ) ;
#29654=ORIENTED_EDGE ( 'NONE', *, *, #31815, .T. ) ;
#29669=AXIS2_PLACEMENT_3D ( 'NONE', #30421, #24423, #54119 ) ;
#29673=ORIENTED_EDGE ( 'NONE', *, *, #40151, .T. ) ;
#29693=ORIENTED_EDGE ( 'NONE', *, *, #15029, .F. ) ;
#29698=CARTESIAN_POINT ( 'NONE',  ( -12.50000000000000000, -107.5000000000000000, 2.500000000000000000 ) ) ;
#29713=DIRECTION ( 'NONE',  ( 0.9435911131814402886, -0.3311129884571281101, 0.000000000000000000 ) ) ;
#29721=VERTEX_POINT ( 'NONE', #36294 ) ;
#29732=DIRECTION ( 'NONE',  ( 0.3090169943749573878, -0.9510565162951503115, 0.000000000000000000 ) ) ;
#29736=ORIENTED_EDGE ( 'NONE', *, *, #28414, .F. ) ;
#29738=ORIENTED_EDGE ( 'NONE', *, *, #5274, .F. ) ;
#29762=EDGE_LOOP ( 'NONE', ( #52820, #28277, #17961, #10990 ) ) ;
#29781=VECTOR ( 'NONE', #60034, 1000.000000000000000 ) ;
#29783=DIRECTION ( 'NONE',  ( 0.9730327541852497042, -0.2306669878475622604, 0.000000000000000000 ) ) ;
#29808=CARTESIAN_POINT ( 'NONE',  ( 12.69589495141918611, -96.69089767102708777, 2.500000000000000000 ) ) ;
#29829=CARTESIAN_POINT ( 'NONE',  ( -0.9515373497862389396, -96.47140937769621871, 5.500000000000000000 ) ) ;
#29854=EDGE_CURVE ( 'NONE', #70242, #63158, #47582, .T. ) ;
#29858=VECTOR ( 'NONE', #72843, 1000.000000000000000 ) ;
#29862=LINE ( 'NONE', #18225, #9845 ) ;
#29878=DIRECTION ( 'NONE',  ( -0.000000000000000000, -0.000000000000000000, -1.000000000000000000 ) ) ;
#29880=FACE_OUTER_BOUND ( 'NONE', #16959, .T. ) ;
#29899=VECTOR ( 'NONE', #12707, 1000.000000000000227 ) ;
#29912=PLANE ( 'NONE',  #71020 ) ;
#29926=CARTESIAN_POINT ( 'NONE',  ( 26.47460221209471598, -121.8961639463267090, 2.500000000000000000 ) ) ;
#29978=ORIENTED_EDGE ( 'NONE', *, *, #64365, .T. ) ;
#30000=VECTOR ( 'NONE', #66022, 1000.000000000000000 ) ;
#30008=FACE_OUTER_BOUND ( 'NONE', #40924, .T. ) ;
#30009=CARTESIAN_POINT ( 'NONE',  ( 12.50000000000000000, -132.5000000000000000, -2.500000000000000000 ) ) ;
#30034=VERTEX_POINT ( 'NONE', #29352 ) ;
#30043=VERTEX_POINT ( 'NONE', #47037 ) ;
#30051=VECTOR ( 'NONE', #7627, 1000.000000000000000 ) ;
#30162=LINE ( 'NONE', #34330, #58348 ) ;
#30178=CARTESIAN_POINT ( 'NONE',  ( 3.429551818649054340, -146.3199197248623875, 5.500000000000000000 ) ) ;
#30188=LINE ( 'NONE', #19278, #28656 ) ;
#30226=VERTEX_POINT ( 'NONE', #54520 ) ;
#30237=VECTOR ( 'NONE', #8530, 1000.000000000000000 ) ;
#30281=DIRECTION ( 'NONE',  ( -0.9730327541852491491, 0.2306669878475648139, 0.000000000000000000 ) ) ;
#30286=EDGE_CURVE ( 'NONE', #17504, #56961, #30460, .T. ) ;
#30353=FACE_OUTER_BOUND ( 'NONE', #58114, .T. ) ;
#30377=EDGE_CURVE ( 'NONE', #55006, #23530, #54158, .T. ) ;
#30396=ORIENTED_EDGE ( 'NONE', *, *, #67291, .F. ) ;
#30399=DIRECTION ( 'NONE',  ( 0.6862798483830533369, 0.7273375899149812085, -0.000000000000000000 ) ) ;
#30416=VERTEX_POINT ( 'NONE', #39461 ) ;
#30421=CARTESIAN_POINT ( 'NONE',  ( 0.000000000000000000, -120.0000000000000000, -2.500000000000000000 ) ) ;
#30460=LINE ( 'NONE', #25937, #28658 ) ;
#30474=EDGE_CURVE ( 'NONE', #31369, #19022, #73280, .T. ) ;
#30480=PLANE ( 'NONE',  #19935 ) ;
#30496=DIRECTION ( 'NONE',  ( -0.000000000000000000, -0.000000000000000000, -1.000000000000000000 ) ) ;
#30512=DIRECTION ( 'NONE',  ( -0.8774505977381978905, -0.4796670183876304283, 0.000000000000000000 ) ) ;
#30516=DIRECTION ( 'NONE',  ( 0.000000000000000000, 0.000000000000000000, 1.000000000000000000 ) ) ;
#30531=CARTESIAN_POINT ( 'NONE',  ( 0.7195005275814480017, -121.3161758966073052, 2.500000000000000000 ) ) ;
#30601=DIRECTION ( 'NONE',  ( -0.000000000000000000, -0.000000000000000000, -1.000000000000000000 ) ) ;
#30615=EDGE_CURVE ( 'NONE', #11307, #59498, #386, .T. ) ;
#30619=EDGE_CURVE ( 'NONE', #43631, #38411, #23282, .T. ) ;
#30635=VECTOR ( 'NONE', #60321, 1000.000000000000000 ) ;
#30678=EDGE_CURVE ( 'NONE', #55143, #31960, #34182, .T. ) ;
#30683=CARTESIAN_POINT ( 'NONE',  ( 25.81725066941077529, -113.8380548628854854, 5.500000000000000000 ) ) ;
#30718=EDGE_LOOP ( 'NONE', ( #56441, #55182, #57050, #60279 ) ) ;
#30731=DIRECTION ( 'NONE',  ( -0.000000000000000000, -0.000000000000000000, -1.000000000000000000 ) ) ;
#30767=AXIS2_PLACEMENT_3D ( 'NONE', #22551, #44372, #39854 ) ;
#30774=ADVANCED_FACE ( 'NONE', ( #70583 ), #64243, .F. ) ;
#30782=ORIENTED_EDGE ( 'NONE', *, *, #23402, .T. ) ;
#30785=ADVANCED_FACE ( 'NONE', ( #42051 ), #37148, .T. ) ;
#30788=FACE_BOUND ( 'NONE', #34757, .T. ) ;
#30792=CARTESIAN_POINT ( 'NONE',  ( -4.653126046682595884, -146.1313684676804314, 5.500000000000000000 ) ) ;
#30793=PLANE ( 'NONE',  #16901 ) ;
#30803=EDGE_CURVE ( 'NONE', #55469, #25695, #65717, .T. ) ;
#30813=VECTOR ( 'NONE', #53584, 1000.000000000000000 ) ;
#30821=LINE ( 'NONE', #54511, #50617 ) ;
#30825=EDGE_CURVE ( 'NONE', #12692, #30034, #18723, .T. ) ;
#30830=PLANE ( 'NONE',  #74234 ) ;
#30834=LINE ( 'NONE', #18451, #18853 ) ;
#30852=FACE_BOUND ( 'NONE', #38448, .T. ) ;
#30860=AXIS2_PLACEMENT_3D ( 'NONE', #19731, #42678, #54333 ) ;
#30878=VERTEX_POINT ( 'NONE', #26215 ) ;
#30896=CARTESIAN_POINT ( 'NONE',  ( -1.499592026101402853, -119.9650177866181764, -2.500000000000000000 ) ) ;
#30900=LINE ( 'NONE', #53113, #60743 ) ;
#30935=AXIS2_PLACEMENT_3D ( 'NONE', #58345, #32894, #35047 ) ;
#30945=VECTOR ( 'NONE', #32037, 1000.000000000000000 ) ;
#30951=ORIENTED_EDGE ( 'NONE', *, *, #60031, .F. ) ;
#30979=DIRECTION ( 'NONE',  ( 0.9827303690289279636, 0.1850432970638682395, -0.000000000000000000 ) ) ;
#31042=PLANE ( 'NONE',  #69609 ) ;
#31075=CARTESIAN_POINT ( 'NONE',  ( -16.07206065793331007, -141.0698568150738197, 2.500000000000000000 ) ) ;
#31087=CARTESIAN_POINT ( 'NONE',  ( 23.49916127795269460, -121.5130826919798039, -5.500000000000000000 ) ) ;
#31094=AXIS2_PLACEMENT_3D ( 'NONE', #14259, #37577, #20648 ) ;
#31096=DIRECTION ( 'NONE',  ( 0.000000000000000000, 0.000000000000000000, 1.000000000000000000 ) ) ;
#31097=VECTOR ( 'NONE', #12818, 1000.000000000000000 ) ;
#31108=CARTESIAN_POINT ( 'NONE',  ( 23.49916127795269460, -121.5130826919798039, 5.500000000000000000 ) ) ;
#31127=AXIS2_PLACEMENT_3D ( 'NONE', #32114, #55053, #3582 ) ;
#31151=DIRECTION ( 'NONE',  ( 0.8225049752423786442, 0.5687579148473752566, -0.000000000000000000 ) ) ;
#31158=ADVANCED_FACE ( 'NONE', ( #33583 ), #61808, .F. ) ;
#31187=AXIS2_PLACEMENT_3D ( 'NONE', #9176, #38863, #32099 ) ;
#31201=DIRECTION ( 'NONE',  ( 1.000000000000000000, 0.000000000000000000, 0.000000000000000000 ) ) ;
#31242=LINE ( 'NONE', #64727, #65285 ) ;
#31251=EDGE_CURVE ( 'NONE', #16009, #19127, #28780, .T. ) ;
#31257=DIRECTION ( 'NONE',  ( -0.7273375899149793211, 0.6862798483830554463, 0.000000000000000000 ) ) ;
#31272=CARTESIAN_POINT ( 'NONE',  ( 21.85433023846371370, -135.0628101570779620, 5.500000000000000000 ) ) ;
#31290=ORIENTED_EDGE ( 'NONE', *, *, #40419, .T. ) ;
#31305=CARTESIAN_POINT ( 'NONE',  ( 16.30584220631899228, -140.9432449716519784, 5.500000000000000000 ) ) ;
#31337=ORIENTED_EDGE ( 'NONE', *, *, #5800, .T. ) ;
#31350=CARTESIAN_POINT ( 'NONE',  ( -22.53294031248082163, -134.0273518838794757, -5.500000000000000000 ) ) ;
#31369=VERTEX_POINT ( 'NONE', #61384 ) ;
#31370=AXIS2_PLACEMENT_3D ( 'NONE', #37799, #8481, #31394 ) ;
#31374=DIRECTION ( 'NONE',  ( -0.000000000000000000, -0.000000000000000000, -1.000000000000000000 ) ) ;
#31383=FACE_OUTER_BOUND ( 'NONE', #6244, .T. ) ;
#31394=DIRECTION ( 'NONE',  ( -0.7273375899149793211, 0.6862798483830554463, 0.000000000000000000 ) ) ;
#31416=VECTOR ( 'NONE', #2915, 1000.000000000000000 ) ;
#31448=PLANE ( 'NONE',  #19387 ) ;
#31458=VERTEX_POINT ( 'NONE', #51195 ) ;
#31471=CIRCLE ( 'NONE', #7443, 32.50000000000000000 ) ;
#31489=ADVANCED_FACE ( 'NONE', ( #34275 ), #18106, .T. ) ;
#31490=DIRECTION ( 'NONE',  ( 0.1850432970638656860, -0.9827303690289285187, 0.000000000000000000 ) ) ;
#31517=CARTESIAN_POINT ( 'NONE',  ( -15.44521549751111422, -137.7748507232956001, 5.500000000000000000 ) ) ;
#31529=VERTEX_POINT ( 'NONE', #28631 ) ;
#31557=LINE ( 'NONE', #1931, #68458 ) ;
#31558=DIRECTION ( 'NONE',  ( -0.3853207896976523772, 0.9227826878668550226, 0.000000000000000000 ) ) ;
#31565=LINE ( 'NONE', #1939, #38657 ) ;
#31597=ORIENTED_EDGE ( 'NONE', *, *, #63766, .F. ) ;
#31604=PLANE ( 'NONE',  #47312 ) ;
#31608=VERTEX_POINT ( 'NONE', #49896 ) ;
#31616=ORIENTED_EDGE ( 'NONE', *, *, #22568, .F. ) ;
#31620=DIRECTION ( 'NONE',  ( -0.3311129884571281101, -0.9435911131814402886, 0.000000000000000000 ) ) ;
#31636=EDGE_LOOP ( 'NONE', ( #53365, #16729, #5320, #13114 ) ) ;
#31649=PLANE ( 'NONE',  #14465 ) ;
#31650=CARTESIAN_POINT ( 'NONE',  ( 26.09152095774781799, -124.8716048804687375, 5.500000000000000000 ) ) ;
#31654=FACE_OUTER_BOUND ( 'NONE', #45974, .T. ) ;
#31693=ORIENTED_EDGE ( 'NONE', *, *, #74029, .T. ) ;
#31734=VECTOR ( 'NONE', #26760, 1000.000000000000114 ) ;
#31759=EDGE_CURVE ( 'NONE', #46309, #31608, #49166, .T. ) ;
#31782=CARTESIAN_POINT ( 'NONE',  ( 20.85212586905262100, -130.9402397935870965, -5.500000000000000000 ) ) ;
#31815=EDGE_CURVE ( 'NONE', #69665, #6591, #38638, .T. ) ;
#31869=ORIENTED_EDGE ( 'NONE', *, *, #48323, .T. ) ;
#31908=FACE_BOUND ( 'NONE', #60208, .T. ) ;
#31922=LINE ( 'NONE', #55974, #15846 ) ;
#31926=FACE_OUTER_BOUND ( 'NONE', #25181, .T. ) ;
#31960=VERTEX_POINT ( 'NONE', #29926 ) ;
#31970=VERTEX_POINT ( 'NONE', #41222 ) ;
#32027=CARTESIAN_POINT ( 'NONE',  ( -30.50000000000000000, -120.0000000000000000, -2.500000000000000000 ) ) ;
#32037=DIRECTION ( 'NONE',  ( -0.000000000000000000, -0.000000000000000000, -1.000000000000000000 ) ) ;
#32042=CARTESIAN_POINT ( 'NONE',  ( -13.05994868825747446, -139.5943292883446532, 5.500000000000000000 ) ) ;
#32099=DIRECTION ( 'NONE',  ( 1.000000000000000000, 0.000000000000000000, 0.000000000000000000 ) ) ;
#32114=CARTESIAN_POINT ( 'NONE',  ( 16.84844760790522855, -103.5491698323862124, 5.500000000000000000 ) ) ;
#32117=CARTESIAN_POINT ( 'NONE',  ( 19.12409105625795291, -101.5943176906707919, 5.500000000000000000 ) ) ;
#32128=CARTESIAN_POINT ( 'NONE',  ( 0.000000000000000000, -120.0000000000000000, 2.500000000000000000 ) ) ;
#32181=LINE ( 'NONE', #48743, #4621 ) ;
#32182=DIRECTION ( 'NONE',  ( -0.000000000000000000, -0.000000000000000000, -1.000000000000000000 ) ) ;
#32201=FACE_OUTER_BOUND ( 'NONE', #57694, .T. ) ;
#32230=EDGE_LOOP ( 'NONE', ( #31337, #19346, #25430, #13926 ) ) ;
#32260=LINE ( 'NONE', #72486, #51347 ) ;
#32265=ORIENTED_EDGE ( 'NONE', *, *, #21102, .T. ) ;
#32280=VECTOR ( 'NONE', #34374, 1000.000000000000114 ) ;
#32281=CARTESIAN_POINT ( 'NONE',  ( -22.67106064244953245, -113.6342314410295842, -5.500000000000000000 ) ) ;
#32291=LINE ( 'NONE', #43245, #48120 ) ;
#32294=FACE_OUTER_BOUND ( 'NONE', #14818, .T. ) ;
#32339=ORIENTED_EDGE ( 'NONE', *, *, #54896, .T. ) ;
#32382=LINE ( 'NONE', #14365, #44309 ) ;
#32393=DIRECTION ( 'NONE',  ( -0.000000000000000000, -0.000000000000000000, -1.000000000000000000 ) ) ;
#32400=DIRECTION ( 'NONE',  ( 0.5200609990132993854, 0.8541291221503275466, -0.000000000000000000 ) ) ;
#32401=CARTESIAN_POINT ( 'NONE',  ( -20.30386590532152979, -102.9045904027214959, -5.500000000000000000 ) ) ;
#32451=ORIENTED_EDGE ( 'NONE', *, *, #73476, .T. ) ;
#32467=CARTESIAN_POINT ( 'NONE',  ( 0.000000000000000000, -120.0000000000000000, 2.500000000000000000 ) ) ;
#32480=LINE ( 'NONE', #42307, #59552 ) ;
#32497=CARTESIAN_POINT ( 'NONE',  ( 26.28306158492127764, -123.3838844133976522, -2.500000000000000000 ) ) ;
#32519=ORIENTED_EDGE ( 'NONE', *, *, #58091, .T. ) ;
#32523=VECTOR ( 'NONE', #20480, 1000.000000000000000 ) ;
#32527=LINE ( 'NONE', #43835, #11673 ) ;
#32535=ORIENTED_EDGE ( 'NONE', *, *, #51, .T. ) ;
#32557=EDGE_CURVE ( 'NONE', #19049, #29007, #48981, .T. ) ;
#32576=STYLED_ITEM ( 'NONE', ( #35470 ), #28332 ) ;
#32594=LINE ( 'NONE', #4054, #6995 ) ;
#32596=VERTEX_POINT ( 'NONE', #71539 ) ;
#32606=ADVANCED_FACE ( 'NONE', ( #5004 ), #74138, .F. ) ;
#32611=EDGE_LOOP ( 'NONE', ( #20804, #58060, #8043, #10341 ) ) ;
#32619=ORIENTED_EDGE ( 'NONE', *, *, #40158, .F. ) ;
#32696=LINE ( 'NONE', #26330, #52367 ) ;
#32705=PLANE ( 'NONE',  #54904 ) ;
#32708=DIRECTION ( 'NONE',  ( -0.1045284632676436315, -0.9945218953682742891, 0.000000000000000000 ) ) ;
#32714=ORIENTED_EDGE ( 'NONE', *, *, #65201, .F. ) ;
#32737=ORIENTED_EDGE ( 'NONE', *, *, #61397, .T. ) ;
#32747=LINE ( 'NONE', #65511, #49930 ) ;
#32751=CIRCLE ( 'NONE', #69992, 30.50000000000000000 ) ;
#32752=VERTEX_POINT ( 'NONE', #39198 ) ;
#32794=AXIS2_PLACEMENT_3D ( 'NONE', #8265, #8647, #31558 ) ;
#32796=VECTOR ( 'NONE', #48501, 1000.000000000000114 ) ;
#32864=DIRECTION ( 'NONE',  ( -0.9038112904824853189, 0.4279312458752977943, 0.000000000000000000 ) ) ;
#32879=ORIENTED_EDGE ( 'NONE', *, *, #4776, .T. ) ;
#32894=DIRECTION ( 'NONE',  ( -0.02332147558787674158, -0.9997280174009349762, 0.000000000000000000 ) ) ;
#32896=ADVANCED_FACE ( 'NONE', ( #70707, #9046, #42526, #59822, #64722, #24858, #13934, #20327, #66209, #41778, #65468, #8311, #3431, #30852, #36137, #59085, #19578 ), #14684, .T. ) ;
#32941=DIRECTION ( 'NONE',  ( -0.000000000000000000, -0.000000000000000000, 1.000000000000000000 ) ) ;
#32943=EDGE_CURVE ( 'NONE', #15838, #29293, #70332, .T. ) ;
#32960=ORIENTED_EDGE ( 'NONE', *, *, #23667, .F. ) ;
#32962=VECTOR ( 'NONE', #42245, 1000.000000000000000 ) ;
#32966=VECTOR ( 'NONE', #35664, 1000.000000000000000 ) ;
#32970=CARTESIAN_POINT ( 'NONE',  ( 12.50000000000000000, -107.5000000000000000, 2.500000000000000000 ) ) ;
#32975=ORIENTED_EDGE ( 'NONE', *, *, #45798, .T. ) ;
#32982=CARTESIAN_POINT ( 'NONE',  ( -12.50000000000000000, -132.5000000000000000, 2.500000000000000000 ) ) ;
#33024=ORIENTED_EDGE ( 'NONE', *, *, #3529, .F. ) ;
#33027=APPLICATION_CONTEXT ( 'automotive_design' ) ;
#33031=ORIENTED_EDGE ( 'NONE', *, *, #32943, .T. ) ;
#33032=CARTESIAN_POINT ( 'NONE',  ( 13.83832728059186046, -142.6495187161941089, 5.500000000000000000 ) ) ;
#33066=VERTEX_POINT ( 'NONE', #26339 ) ;
#33094=ORIENTED_EDGE ( 'NONE', *, *, #26387, .T. ) ;
#33101=ORIENTED_EDGE ( 'NONE', *, *, #40151, .F. ) ;
#33126=FACE_OUTER_BOUND ( 'NONE', #47139, .T. ) ;
#33132=PLANE ( 'NONE',  #62676 ) ;
#33135=ORIENTED_EDGE ( 'NONE', *, *, #18241, .T. ) ;
#33148=DIRECTION ( 'NONE',  ( 0.02332147558787671729, 0.9997280174009349762, -0.000000000000000000 ) ) ;
#33176=VERTEX_POINT ( 'NONE', #35319 ) ;
#33178=ADVANCED_FACE ( 'NONE', ( #63904 ), #57517, .F. ) ;
#33220=CARTESIAN_POINT ( 'NONE',  ( 0.000000000000000000, -120.0000000000000000, 2.500000000000000000 ) ) ;
#33228=CARTESIAN_POINT ( 'NONE',  ( 0.000000000000000000, -89.50000000000000000, -5.500000000000000000 ) ) ;
#33229=LINE ( 'NONE', #55809, #12642 ) ;
#33245=ADVANCED_FACE ( 'NONE', ( #22562 ), #45507, .F. ) ;
#33249=VECTOR ( 'NONE', #860, 1000.000000000000000 ) ;
#33287=ORIENTED_EDGE ( 'NONE', *, *, #22533, .F. ) ;
#33298=LINE ( 'NONE', #56254, #24139 ) ;
#33334=EDGE_CURVE ( 'NONE', #50088, #31458, #41688, .T. ) ;
#33358=ORIENTED_EDGE ( 'NONE', *, *, #71967, .T. ) ;
#33381=DIRECTION ( 'NONE',  ( -0.3311129884571281101, -0.9435911131814402886, 0.000000000000000000 ) ) ;
#33390=VERTEX_POINT ( 'NONE', #37174 ) ;
#33415=EDGE_CURVE ( 'NONE', #25489, #24434, #48806, .T. ) ;
#33500=CARTESIAN_POINT ( 'NONE',  ( -20.30386590532152979, -102.9045904027214959, 5.500000000000000000 ) ) ;
#33504=AXIS2_PLACEMENT_3D ( 'NONE', #46466, #29524, #12248 ) ;
#33527=ORIENTED_EDGE ( 'NONE', *, *, #57321, .F. ) ;
#33532=ORIENTED_EDGE ( 'NONE', *, *, #12645, .T. ) ;
#33545=DIRECTION ( 'NONE',  ( 0.4279312458752976833, 0.9038112904824853189, -0.000000000000000000 ) ) ;
#33555=CARTESIAN_POINT ( 'NONE',  ( -114.1267819554185365, -82.91796067500661138, 5.500000000000000000 ) ) ;
#33573=VECTOR ( 'NONE', #55916, 1000.000000000000000 ) ;
#33583=FACE_OUTER_BOUND ( 'NONE', #18742, .T. ) ;
#33608=CARTESIAN_POINT ( 'NONE',  ( 2.117611129180199558, -93.54218975225703048, 5.500000000000000000 ) ) ;
#33625=CARTESIAN_POINT ( 'NONE',  ( 23.41451323550360186, -132.5004227906269989, 2.500000000000000000 ) ) ;
#33635=EDGE_CURVE ( 'NONE', #24993, #62465, #67217, .T. ) ;
#33636=CARTESIAN_POINT ( 'NONE',  ( 12.69589495141918611, -96.69089767102708777, 5.500000000000000000 ) ) ;
#33652=ORIENTED_EDGE ( 'NONE', *, *, #9173, .T. ) ;
#33676=EDGE_CURVE ( 'NONE', #42185, #7680, #18939, .T. ) ;
#33691=ADVANCED_FACE ( 'NONE', ( #53171 ), #16457, .T. ) ;
#33703=FACE_OUTER_BOUND ( 'NONE', #3981, .T. ) ;
#33715=DIRECTION ( 'NONE',  ( -0.000000000000000000, -0.000000000000000000, -1.000000000000000000 ) ) ;
#33718=AXIS2_PLACEMENT_3D ( 'NONE', #53588, #13726, #6266 ) ;
#33731=EDGE_CURVE ( 'NONE', #39126, #14221, #70072, .T. ) ;
#33733=CARTESIAN_POINT ( 'NONE',  ( 3.429551818649054340, -146.3199197248623875, 5.500000000000000000 ) ) ;
#33736=ORIENTED_EDGE ( 'NONE', *, *, #50560, .T. ) ;
#33740=LINE ( 'NONE', #61947, #14717 ) ;
#33746=DIRECTION ( 'NONE',  ( -0.000000000000000000, -0.000000000000000000, -1.000000000000000000 ) ) ;
#33747=ORIENTED_EDGE ( 'NONE', *, *, #38622, .T. ) ;
#33763=ORIENTED_EDGE ( 'NONE', *, *, #54812, .F. ) ;
#33769=CARTESIAN_POINT ( 'NONE',  ( -23.30023580412278505, -123.4057321492263384, 5.500000000000000000 ) ) ;
#33798=DIRECTION ( 'NONE',  ( 0.9918136447140104561, -0.1276937514489679681, 0.000000000000000000 ) ) ;
#33804=LINE ( 'NONE', #44726, #63891 ) ;
#33805=CARTESIAN_POINT ( 'NONE',  ( -8.826826895187510402, -94.96827758698185562, 5.500000000000000000 ) ) ;
#33854=LINE ( 'NONE', #6411, #17412 ) ;
#33901=CARTESIAN_POINT ( 'NONE',  ( 26.47460221209471953, -121.8961639463267090, -2.500000000000000000 ) ) ;
#33903=DIRECTION ( 'NONE',  ( 0.9580045777625458836, 0.2867529058022011412, 0.000000000000000000 ) ) ;
#33922=DIRECTION ( 'NONE',  ( -0.9038112904824853189, 0.4279312458752976833, 0.000000000000000000 ) ) ;
#33943=VERTEX_POINT ( 'NONE', #4272 ) ;
#34015=EDGE_LOOP ( 'NONE', ( #33287, #62264, #63997, #57039 ) ) ;
#34030=AXIS2_PLACEMENT_3D ( 'NONE', #46883, #29194, #13018 ) ;
#34066=PLANE ( 'NONE',  #1765 ) ;
#34070=VECTOR ( 'NONE', #30512, 1000.000000000000000 ) ;
#34077=LINE ( 'NONE', #23183, #5264 ) ;
#34094=VECTOR ( 'NONE', #20233, 1000.000000000000000 ) ;
#34120=DIRECTION ( 'NONE',  ( 0.9135454576426059736, -0.4067366430757887730, 0.000000000000000000 ) ) ;
#34169=PLANE ( 'NONE',  #61414 ) ;
#34182=LINE ( 'NONE', #753, #1199 ) ;
#34184=CARTESIAN_POINT ( 'NONE',  ( -22.53294031248082163, -134.0273518838794757, 5.500000000000000000 ) ) ;
#34185=ORIENTED_EDGE ( 'NONE', *, *, #47515, .T. ) ;
#34205=DIRECTION ( 'NONE',  ( -0.6516173805718067369, 0.7585478161175716050, 0.000000000000000000 ) ) ;
#34211=ORIENTED_EDGE ( 'NONE', *, *, #29282, .F. ) ;
#34216=LINE ( 'NONE', #56791, #21376 ) ;
#34223=DIRECTION ( 'NONE',  ( 0.7273375899149812085, -0.6862798483830533369, 0.000000000000000000 ) ) ;
#34240=EDGE_LOOP ( 'NONE', ( #3977, #70500, #35436, #16001 ) ) ;
#34250=LINE ( 'NONE', #24100, #17579 ) ;
#34267=CARTESIAN_POINT ( 'NONE',  ( 70.53423027509757048, -217.0820393249931044, -5.500000000000000000 ) ) ;
#34275=FACE_OUTER_BOUND ( 'NONE', #218, .T. ) ;
#34278=DIRECTION ( 'NONE',  ( -0.9435911131814395114, 0.3311129884571304971, 0.000000000000000000 ) ) ;
#34279=CARTESIAN_POINT ( 'NONE',  ( 9.984461079971730157, -95.40710393340120277, 2.500000000000000000 ) ) ;
#34286=LINE ( 'NONE', #22275, #897 ) ;
#34293=EDGE_LOOP ( 'NONE', ( #5005, #50393, #57705, #51413 ) ) ;
#34299=VERTEX_POINT ( 'NONE', #60221 ) ;
#34301=VECTOR ( 'NONE', #74272, 1000.000000000000000 ) ;
#34311=SHAPE_DEFINITION_REPRESENTATION ( #44618, #23897 ) ;
#34330=CARTESIAN_POINT ( 'NONE',  ( -8.826826895187510402, -94.96827758698185562, -5.500000000000000000 ) ) ;
#34349=FACE_OUTER_BOUND ( 'NONE', #30718, .T. ) ;
#34351=PLANE ( 'NONE',  #62224 ) ;
#34357=EDGE_CURVE ( 'NONE', #57544, #33176, #21435, .T. ) ;
#34374=DIRECTION ( 'NONE',  ( 0.9827303690289279636, 0.1850432970638681840, 0.000000000000000000 ) ) ;
#34438=CARTESIAN_POINT ( 'NONE',  ( -6.880223345695647197, -142.5202692415819854, -2.500000000000000000 ) ) ;
#34440=DIRECTION ( 'NONE',  ( -0.8225049752423776450, -0.5687579148473765889, 0.000000000000000000 ) ) ;
#34462=VECTOR ( 'NONE', #9741, 1000.000000000000114 ) ;
#34511=EDGE_LOOP ( 'NONE', ( #62037, #70733, #42996, #29513 ) ) ;
#34514=VERTEX_POINT ( 'NONE', #64 ) ;
#34551=CARTESIAN_POINT ( 'NONE',  ( -11.59517495878806947, -96.12423995607481686, 2.500000000000000000 ) ) ;
#34579=DIRECTION ( 'NONE',  ( 0.9435911131814398445, -0.3311129884571295534, 0.000000000000000000 ) ) ;
#34582=LINE ( 'NONE', #46244, #16685 ) ;
#34591=EDGE_LOOP ( 'NONE', ( #54944, #26559, #22501, #24079 ) ) ;
#34595=ORIENTED_EDGE ( 'NONE', *, *, #565, .T. ) ;
#34664=ORIENTED_EDGE ( 'NONE', *, *, #66110, .T. ) ;
#34694=ORIENTED_EDGE ( 'NONE', *, *, #73298, .T. ) ;
#34721=CARTESIAN_POINT ( 'NONE',  ( 1.192633404626820770, -120.9097392825245407, -2.500000000000000000 ) ) ;
#34733=AXIS2_PLACEMENT_3D ( 'NONE', #3829, #54939, #60597 ) ;
#34757=EDGE_LOOP ( 'NONE', ( #35050, #42924, #67312, #52090 ) ) ;
#34775=EDGE_LOOP ( 'NONE', ( #65244, #44390, #46137, #62735 ) ) ;
#34819=AXIS2_PLACEMENT_3D ( 'NONE', #22039, #44981, #10760 ) ;
#34834=LINE ( 'NONE', #29170, #21408 ) ;
#34836=VERTEX_POINT ( 'NONE', #64810 ) ;
#34880=VERTEX_POINT ( 'NONE', #53885 ) ;
#34899=ORIENTED_EDGE ( 'NONE', *, *, #60762, .F. ) ;
#34905=ORIENTED_EDGE ( 'NONE', *, *, #2758, .F. ) ;
#34947=CIRCLE ( 'NONE', #12085, 35.50000000000000711 ) ;
#34951=VERTEX_POINT ( 'NONE', #53866 ) ;
#34980=DIRECTION ( 'NONE',  ( -0.9997280174009349762, 0.02332147558787674504, 0.000000000000000000 ) ) ;
#35010=CARTESIAN_POINT ( 'NONE',  ( -23.97194136764370853, -131.3950000906648938, 2.500000000000000000 ) ) ;
#35014=AXIS2_PLACEMENT_3D ( 'NONE', #72248, #59138, #9102 ) ;
#35020=DIRECTION ( 'NONE',  ( -0.8225049752423776450, -0.5687579148473765889, 0.000000000000000000 ) ) ;
#35028=( NAMED_UNIT ( * ) PLANE_ANGLE_UNIT ( ) SI_UNIT ( $, .RADIAN. ) );
#35029=VERTEX_POINT ( 'NONE', #50348 ) ;
#35033=EDGE_LOOP ( 'NONE', ( #29576, #71959, #70611, #5451 ) ) ;
#35047=DIRECTION ( 'NONE',  ( 0.9997280174009349762, -0.02332147558787674158, 0.000000000000000000 ) ) ;
#35050=ORIENTED_EDGE ( 'NONE', *, *, #68329, .F. ) ;
#35100=CARTESIAN_POINT ( 'NONE',  ( -22.53294031248082163, -134.0273518838794757, 5.500000000000000000 ) ) ;
#35140=EDGE_LOOP ( 'NONE', ( #37939, #29978, #72735, #69983 ) ) ;
#35151=CARTESIAN_POINT ( 'NONE',  ( 19.29194287201271862, -133.5026271600380880, 5.500000000000000000 ) ) ;
#35168=EDGE_CURVE ( 'NONE', #2800, #65294, #40557, .T. ) ;
#35174=CARTESIAN_POINT ( 'NONE',  ( -0.8815729230226008184, -93.47222532549339746, 5.500000000000000000 ) ) ;
#35215=CYLINDRICAL_SURFACE ( 'NONE', #14769, 30.50000000000000000 ) ;
#35221=DIRECTION ( 'NONE',  ( 1.000000000000000000, 0.000000000000000000, 0.000000000000000000 ) ) ;
#35224=VERTEX_POINT ( 'NONE', #58581 ) ;
#35251=LINE ( 'NONE', #1087, #48607 ) ;
#35264=FACE_OUTER_BOUND ( 'NONE', #55883, .T. ) ;
#35274=FACE_OUTER_BOUND ( 'NONE', #53156, .T. ) ;
#35275=VECTOR ( 'NONE', #39766, 1000.000000000000000 ) ;
#35297=ORIENTED_EDGE ( 'NONE', *, *, #27249, .F. ) ;
#35307=ADVANCED_FACE ( 'NONE', ( #64599 ), #69859, .T. ) ;
#35311=ORIENTED_EDGE ( 'NONE', *, *, #3994, .F. ) ;
#35319=CARTESIAN_POINT ( 'NONE',  ( 21.85433023846372436, -135.0628101570779620, 2.500000000000000000 ) ) ;
#35335=ORIENTED_EDGE ( 'NONE', *, *, #4072, .T. ) ;
#35379=AXIS2_PLACEMENT_3D ( 'NONE', #2635, #31151, #37917 ) ;
#35384=ADVANCED_FACE ( 'NONE', ( #58967 ), #13816, .F. ) ;
#35394=VECTOR ( 'NONE', #60994, 1000.000000000000114 ) ;
#35395=CARTESIAN_POINT ( 'NONE',  ( 0.000000000000000000, 0.000000000000000000, 5.500000000000000000 ) ) ;
#35427=DIRECTION ( 'NONE',  ( 0.08130631524009970801, -0.9966891607226786576, 0.000000000000000000 ) ) ;
#35436=ORIENTED_EDGE ( 'NONE', *, *, #13418, .T. ) ;
#35440=CARTESIAN_POINT ( 'NONE',  ( 9.984461079971730157, -95.40710393340120277, -5.500000000000000000 ) ) ;
#35454=CARTESIAN_POINT ( 'NONE',  ( 25.81725066941077529, -113.8380548628854854, -2.500000000000000444 ) ) ;
#35461=DIRECTION ( 'NONE',  ( 0.8774505977381978905, 0.4796670183876304283, 0.000000000000000000 ) ) ;
#35464=DIRECTION ( 'NONE',  ( -0.000000000000000000, -0.000000000000000000, 1.000000000000000000 ) ) ;
#35470=PRESENTATION_STYLE_ASSIGNMENT (( #12533 ) ) ;
#35506=DIRECTION ( 'NONE',  ( -0.8541291221503261033, 0.5200609990133016058, 0.000000000000000000 ) ) ;
#35515=DIRECTION ( 'NONE',  ( -0.08130631524010122069, 0.9966891607226784355, 0.000000000000000000 ) ) ;
#35532=DIRECTION ( 'NONE',  ( 0.9038112904824853189, -0.4279312458752977388, 0.000000000000000000 ) ) ;
#35545=DIRECTION ( 'NONE',  ( 0.9966891607226786576, 0.08130631524009862554, 0.000000000000000000 ) ) ;
#35559=VECTOR ( 'NONE', #64675, 1000.000000000000000 ) ;
#35584=CARTESIAN_POINT ( 'NONE',  ( -4.653126046682595884, -146.1313684676804314, -5.500000000000000000 ) ) ;
#35590=CARTESIAN_POINT ( 'NONE',  ( -18.24502636017238899, -100.7225776329765665, -5.500000000000000000 ) ) ;
#35617=EDGE_LOOP ( 'NONE', ( #27158, #50887, #17662, #20051 ) ) ;
#35632=DIRECTION ( 'NONE',  ( 0.2867529058022035837, -0.9580045777625452175, 0.000000000000000000 ) ) ;
#35635=EDGE_CURVE ( 'NONE', #34880, #22108, #11162, .T. ) ;
#35642=DIRECTION ( 'NONE',  ( -0.1276937514489705217, -0.9918136447140101231, 0.000000000000000000 ) ) ;
#35651=DIRECTION ( 'NONE',  ( -0.4796670183876317051, 0.8774505977381972244, 0.000000000000000000 ) ) ;
#35664=DIRECTION ( 'NONE',  ( 0.6516173805718078471, -0.7585478161175706058, 0.000000000000000000 ) ) ;
#35747=CARTESIAN_POINT ( 'NONE',  ( -35.50000000000000711, -120.0000000000000000, -2.500000000000000000 ) ) ;
#35758=VECTOR ( 'NONE', #62237, 1000.000000000000114 ) ;
#35765=DIRECTION ( 'NONE',  ( -0.9730327541852497042, 0.2306669878475622604, 0.000000000000000000 ) ) ;
#35771=AXIS2_PLACEMENT_3D ( 'NONE', #66282, #49337, #72266 ) ;
#35774=ADVANCED_FACE ( 'NONE', ( #6989 ), #29912, .F. ) ;
#35775=ORIENTED_EDGE ( 'NONE', *, *, #1266, .T. ) ;
#35805=EDGE_LOOP ( 'NONE', ( #66591, #33736, #32879, #38394 ) ) ;
#35826=( NAMED_UNIT ( * ) PLANE_ANGLE_UNIT ( ) SI_UNIT ( $, .RADIAN. ) );
#35856=ORIENTED_EDGE ( 'NONE', *, *, #29375, .F. ) ;
#35864=ORIENTED_EDGE ( 'NONE', *, *, #41951, .T. ) ;
#35865=VECTOR ( 'NONE', #41365, 1000.000000000000114 ) ;
#35890=LINE ( 'NONE', #64853, #18153 ) ;
#35894=DIRECTION ( 'NONE',  ( -0.5687579148473752566, 0.8225049752423786442, 0.000000000000000000 ) ) ;
#35895=ADVANCED_FACE ( 'NONE', ( #26126 ), #27225, .F. ) ;
#35899=ORIENTED_EDGE ( 'NONE', *, *, #49841, .T. ) ;
#35909=ADVANCED_FACE ( 'NONE', ( #71986 ), #54346, .F. ) ;
#35935=CIRCLE ( 'NONE', #71932, 30.50000000000000000 ) ;
#35980=CARTESIAN_POINT ( 'NONE',  ( -103.9230484541323705, -180.0000000000004832, 5.500000000000000000 ) ) ;
#35990=ORIENTED_EDGE ( 'NONE', *, *, #19196, .F. ) ;
#35995=CARTESIAN_POINT ( 'NONE',  ( -8.826826895187510402, -94.96827758698185562, 5.500000000000000000 ) ) ;
#36011=CARTESIAN_POINT ( 'NONE',  ( 23.41451323550360186, -132.5004227906269989, -5.500000000000000000 ) ) ;
#36014=LINE ( 'NONE', #31108, #74081 ) ;
#36017=ADVANCED_FACE ( 'NONE', ( #44923 ), #23100, .F. ) ;
#36028=PLANE ( 'NONE',  #64270 ) ;
#36039=VECTOR ( 'NONE', #34278, 1000.000000000000000 ) ;
#36054=EDGE_CURVE ( 'NONE', #33176, #38913, #27613, .T. ) ;
#36083=EDGE_CURVE ( 'NONE', #6231, #44562, #62593, .T. ) ;
#36095=DIRECTION ( 'NONE',  ( -0.9038112904824846527, 0.4279312458752990711, 0.000000000000000000 ) ) ;
#36111=FACE_OUTER_BOUND ( 'NONE', #23677, .T. ) ;
#36128=LINE ( 'NONE', #53790, #9159 ) ;
#36137=FACE_BOUND ( 'NONE', #34591, .T. ) ;
#36139=VECTOR ( 'NONE', #16021, 1000.000000000000000 ) ;
#36153=ORIENTED_EDGE ( 'NONE', *, *, #14094, .F. ) ;
#36166=FACE_OUTER_BOUND ( 'NONE', #24277, .T. ) ;
#36174=DIRECTION ( 'NONE',  ( -0.8541291221503275466, 0.5200609990132993854, 0.000000000000000000 ) ) ;
#36180=MECHANICAL_DESIGN_GEOMETRIC_PRESENTATION_REPRESENTATION('',(#32576),#42256);
#36182=LINE ( 'NONE', #59128, #45884 ) ;
#36196=DIRECTION ( 'NONE',  ( -0.000000000000000000, -0.000000000000000000, -1.000000000000000000 ) ) ;
#36245=ORIENTED_EDGE ( 'NONE', *, *, #47381, .F. ) ;
#36280=CARTESIAN_POINT ( 'NONE',  ( 9.984461079971730157, -95.40710393340120277, 5.500000000000000000 ) ) ;
#36294=CARTESIAN_POINT ( 'NONE',  ( -20.30386590532152979, -102.9045904027214959, -5.500000000000000000 ) ) ;
#36314=EDGE_CURVE ( 'NONE', #2654, #43742, #37709, .T. ) ;
#36318=ORIENTED_EDGE ( 'NONE', *, *, #20646, .F. ) ;
#36328=VERTEX_POINT ( 'NONE', #9860 ) ;
#36343=EDGE_CURVE ( 'NONE', #40406, #55116, #42603, .T. ) ;
#36350=CARTESIAN_POINT ( 'NONE',  ( -15.44521549751111422, -137.7748507232956001, 5.500000000000000000 ) ) ;
#36352=CARTESIAN_POINT ( 'NONE',  ( -12.50000000000000000, -107.5000000000000000, 2.500000000000000000 ) ) ;
#36354=EDGE_LOOP ( 'NONE', ( #18605, #37487, #74245, #2197 ) ) ;
#36355=CARTESIAN_POINT ( 'NONE',  ( -21.33958957442910886, -129.9559990355020034, 5.500000000000000000 ) ) ;
#36367=ORIENTED_EDGE ( 'NONE', *, *, #10881, .T. ) ;
#36375=CARTESIAN_POINT ( 'NONE',  ( 20.07203437053270179, -132.2214334768125354, 2.500000000000000000 ) ) ;
#36377=LINE ( 'NONE', #59324, #46598 ) ;
#36385=CARTESIAN_POINT ( 'NONE',  ( 20.85212586905262100, -130.9402397935870965, 5.500000000000000000 ) ) ;
#36386=ADVANCED_FACE ( 'NONE', ( #60990 ), #15124, .F. ) ;
#36390=VERTEX_POINT ( 'NONE', #9487 ) ;
#36394=CARTESIAN_POINT ( 'NONE',  ( 24.95699195200416654, -110.9640411295978595, 5.500000000000000000 ) ) ;
#36402=ORIENTED_EDGE ( 'NONE', *, *, #14155, .T. ) ;
#36405=EDGE_CURVE ( 'NONE', #52162, #7502, #59904, .T. ) ;
#36411=ORIENTED_EDGE ( 'NONE', *, *, #69944, .F. ) ;
#36433=ORIENTED_EDGE ( 'NONE', *, *, #62141, .F. ) ;
#36481=AXIS2_PLACEMENT_3D ( 'NONE', #8333, #19967, #42922 ) ;
#36484=DIRECTION ( 'NONE',  ( 0.3311129884571280546, 0.9435911131814402886, 0.000000000000000000 ) ) ;
#36504=AXIS2_PLACEMENT_3D ( 'NONE', #53407, #8278, #47756 ) ;
#36512=DIRECTION ( 'NONE',  ( -0.000000000000000000, -0.000000000000000000, -1.000000000000000000 ) ) ;
#36513=ORIENTED_EDGE ( 'NONE', *, *, #5644, .F. ) ;
#36538=CARTESIAN_POINT ( 'NONE',  ( -8.826826895187510402, -94.96827758698185562, 5.500000000000000000 ) ) ;
#36547=EDGE_LOOP ( 'NONE', ( #40173, #52002, #32619, #71331 ) ) ;
#36556=DIRECTION ( 'NONE',  ( 0.08130631524010120681, -0.9966891607226784355, 0.000000000000000000 ) ) ;
#36592=DIRECTION ( 'NONE',  ( 0.02332147558787671729, 0.9997280174009349762, -0.000000000000000000 ) ) ;
#36602=ORIENTED_EDGE ( 'NONE', *, *, #22094, .T. ) ;
#36604=ORIENTED_EDGE ( 'NONE', *, *, #41951, .F. ) ;
#36610=VECTOR ( 'NONE', #1909, 1000.000000000000000 ) ;
#36638=EDGE_LOOP ( 'NONE', ( #67737, #54955, #56994, #28944 ) ) ;
#36641=ORIENTED_EDGE ( 'NONE', *, *, #33676, .F. ) ;
#36679=ADVANCED_FACE ( 'NONE', ( #46305 ), #69233, .F. ) ;
#36684=VECTOR ( 'NONE', #15466, 1000.000000000000114 ) ;
#36709=EDGE_LOOP ( 'NONE', ( #9171, #2372, #37362, #20314 ) ) ;
#36719=DIRECTION ( 'NONE',  ( 0.2306669878475637314, 0.9730327541852493711, -0.000000000000000000 ) ) ;
#36720=DIRECTION ( 'NONE',  ( -0.000000000000000000, -0.000000000000000000, -1.000000000000000000 ) ) ;
#36753=CARTESIAN_POINT ( 'NONE',  ( 21.07894319797337701, -103.8699611390234878, 5.500000000000000000 ) ) ;
#36757=DIRECTION ( 'NONE',  ( 0.9135454576426004225, 0.4067366430758009854, 0.000000000000000000 ) ) ;
#36795=ORIENTED_EDGE ( 'NONE', *, *, #2321, .T. ) ;
#36798=EDGE_LOOP ( 'NONE', ( #42293, #48704, #44686, #65028 ) ) ;
#36809=ORIENTED_EDGE ( 'NONE', *, *, #50689, .T. ) ;
#36813=LINE ( 'NONE', #8630, #4941 ) ;
#36815=EDGE_CURVE ( 'NONE', #3022, #38305, #45863, .T. ) ;
#36839=CARTESIAN_POINT ( 'NONE',  ( 30.50000000000000000, -120.0000000000000000, 5.500000000000000888 ) ) ;
#36898=ADVANCED_FACE ( 'NONE', ( #39093 ), #15786, .F. ) ;
#36903=EDGE_CURVE ( 'NONE', #44417, #56961, #22928, .T. ) ;
#36907=CARTESIAN_POINT ( 'NONE',  ( 13.83832728059186046, -142.6495187161941089, -5.500000000000000000 ) ) ;
#36923=DIRECTION ( 'NONE',  ( -0.08130631524010117905, 0.9966891607226784355, 0.000000000000000000 ) ) ;
#36926=ORIENTED_EDGE ( 'NONE', *, *, #4169, .F. ) ;
#36952=EDGE_CURVE ( 'NONE', #65921, #45237, #48337, .T. ) ;
#36968=FACE_OUTER_BOUND ( 'NONE', #14342, .T. ) ;
#36982=VECTOR ( 'NONE', #42811, 1000.000000000000114 ) ;
#37013=LINE ( 'NONE', #61437, #59513 ) ;
#37079=ORIENTED_EDGE ( 'NONE', *, *, #49071, .T. ) ;
#37080=ORIENTED_EDGE ( 'NONE', *, *, #41427, .F. ) ;
#37081=VERTEX_POINT ( 'NONE', #4722 ) ;
#37106=FACE_OUTER_BOUND ( 'NONE', #28280, .T. ) ;
#37120=PLANE ( 'NONE',  #64147 ) ;
#37148=CYLINDRICAL_SURFACE ( 'NONE', #62401, 35.50000000000000711 ) ;
#37156=AXIS2_PLACEMENT_3D ( 'NONE', #44856, #55379, #9517 ) ;
#37174=CARTESIAN_POINT ( 'NONE',  ( -14.87942725330654348, -141.9795960975983178, -2.500000000000000000 ) ) ;
#37180=LINE ( 'NONE', #31517, #34094 ) ;
#37182=EDGE_LOOP ( 'NONE', ( #46069, #47886, #45780, #15982 ) ) ;
#37190=ORIENTED_EDGE ( 'NONE', *, *, #41163, .F. ) ;
#37203=DIRECTION ( 'NONE',  ( -0.4796670183876317051, 0.8774505977381971134, 0.000000000000000000 ) ) ;
#37207=EDGE_CURVE ( 'NONE', #41508, #34514, #20870, .T. ) ;
#37216=LINE ( 'NONE', #19531, #72283 ) ;
#37234=VECTOR ( 'NONE', #52925, 1000.000000000000000 ) ;
#37240=DIRECTION ( 'NONE',  ( 0.000000000000000000, -1.000000000000000000, 0.000000000000000000 ) ) ;
#37273=DIRECTION ( 'NONE',  ( 0.000000000000000000, 0.000000000000000000, 1.000000000000000000 ) ) ;
#37291=ORIENTED_EDGE ( 'NONE', *, *, #35168, .F. ) ;
#37295=ORIENTED_EDGE ( 'NONE', *, *, #12660, .F. ) ;
#37296=CARTESIAN_POINT ( 'NONE',  ( -17.26469406256017791, -140.1601175325492648, -2.500000000000000444 ) ) ;
#37302=ORIENTED_EDGE ( 'NONE', *, *, #9533, .T. ) ;
#37328=CARTESIAN_POINT ( 'NONE',  ( -32.50000000000000000, -120.0000000000000000, 2.500000000000000000 ) ) ;
#37337=EDGE_CURVE ( 'NONE', #6591, #26875, #27989, .T. ) ;
#37360=EDGE_LOOP ( 'NONE', ( #39560, #37079, #60476, #29643 ) ) ;
#37362=ORIENTED_EDGE ( 'NONE', *, *, #43218, .T. ) ;
#37366=PRODUCT ( 'Sliding Dog Clutch Collar', 'Sliding Dog Clutch Collar', '', ( #51972 ) ) ;
#37371=ADVANCED_FACE ( 'NONE', ( #580 ), #23112, .F. ) ;
#37386=LINE ( 'NONE', #26079, #30635 ) ;
#37402=ADVANCED_FACE ( 'NONE', ( #36968 ), #949, .F. ) ;
#37424=LINE ( 'NONE', #26114, #56104 ) ;
#37440=EDGE_CURVE ( 'NONE', #48661, #11723, #52401, .T. ) ;
#37453=ORIENTED_EDGE ( 'NONE', *, *, #64889, .F. ) ;
#37477=LINE ( 'NONE', #19787, #30237 ) ;
#37487=ORIENTED_EDGE ( 'NONE', *, *, #46762, .F. ) ;
#37495=CARTESIAN_POINT ( 'NONE',  ( 35.50000000000000711, -120.0000000000000000, 5.500000000000000000 ) ) ;
#37507=DIRECTION ( 'NONE',  ( -0.2306669878475648139, -0.9730327541852491491, 0.000000000000000000 ) ) ;
#37520=ADVANCED_FACE ( 'NONE', ( #73005 ), #8768, .F. ) ;
#37521=DIRECTION ( 'NONE',  ( -0.9827303690289285187, -0.1850432970638656860, 0.000000000000000000 ) ) ;
#37534=EDGE_CURVE ( 'NONE', #3726, #26049, #25685, .T. ) ;
#37537=DIRECTION ( 'NONE',  ( -0.3311129884571280546, -0.9435911131814402886, 0.000000000000000000 ) ) ;
#37554=VERTEX_POINT ( 'NONE', #55734 ) ;
#37577=DIRECTION ( 'NONE',  ( -0.7273375899149812085, 0.6862798483830533369, 0.000000000000000000 ) ) ;
#37591=EDGE_CURVE ( 'NONE', #31970, #12223, #44467, .T. ) ;
#37602=AXIS2_PLACEMENT_3D ( 'NONE', #3495, #66989, #72258 ) ;
#37603=LINE ( 'NONE', #20668, #32796 ) ;
#37639=ORIENTED_EDGE ( 'NONE', *, *, #30474, .F. ) ;
#37681=CARTESIAN_POINT ( 'NONE',  ( -26.53422223201112828, -120.6595836127786043, 5.500000000000000000 ) ) ;
#37709=LINE ( 'NONE', #3142, #30945 ) ;
#37720=DIRECTION ( 'NONE',  ( 0.8541291221503265474, -0.5200609990133007177, 0.000000000000000000 ) ) ;
#37728=VERTEX_POINT ( 'NONE', #39937 ) ;
#37730=VERTEX_POINT ( 'NONE', #34279 ) ;
#37755=ADVANCED_FACE ( 'NONE', ( #17364 ), #30480, .F. ) ;
#37763=DIRECTION ( 'NONE',  ( -0.6862798483830533369, -0.7273375899149812085, 0.000000000000000000 ) ) ;
#37782=MANIFOLD_SOLID_BREP ( 'Revolve1', #44012 ) ;
#37789=CARTESIAN_POINT ( 'NONE',  ( -19.90058851926621131, -132.5883508287165853, 5.500000000000000000 ) ) ;
#37799=CARTESIAN_POINT ( 'NONE',  ( -20.30386590532152979, -102.9045904027214959, 5.500000000000000000 ) ) ;
#37810=ORIENTED_EDGE ( 'NONE', *, *, #28203, .T. ) ;
#37848=EDGE_CURVE ( 'NONE', #12223, #2654, #36128, .T. ) ;
#37887=EDGE_CURVE ( 'NONE', #27626, #26875, #15044, .T. ) ;
#37890=VECTOR ( 'NONE', #65550, 1000.000000000000000 ) ;
#37902=CARTESIAN_POINT ( 'NONE',  ( -11.59517495878806947, -96.12423995607481686, 5.500000000000000000 ) ) ;
#37915=DIRECTION ( 'NONE',  ( 0.2867529058022035837, -0.9580045777625452175, 0.000000000000000000 ) ) ;
#37917=DIRECTION ( 'NONE',  ( -0.5687579148473752566, 0.8225049752423786442, 0.000000000000000000 ) ) ;
#37930=CARTESIAN_POINT ( 'NONE',  ( 23.11608002360578240, -124.4885236261218182, 5.500000000000000000 ) ) ;
#37939=ORIENTED_EDGE ( 'NONE', *, *, #59021, .F. ) ;
#37964=EDGE_CURVE ( 'NONE', #32596, #28941, #32696, .T. ) ;
#37973=VECTOR ( 'NONE', #7893, 1000.000000000000227 ) ;
#38006=ORIENTED_EDGE ( 'NONE', *, *, #24630, .F. ) ;
#38008=VERTEX_POINT ( 'NONE', #45119 ) ;
#38025=ORIENTED_EDGE ( 'NONE', *, *, #47419, .F. ) ;
#38026=DIRECTION ( 'NONE',  ( -0.000000000000000000, -0.000000000000000000, -1.000000000000000000 ) ) ;
#38039=PLANE ( 'NONE',  #39709 ) ;
#38053=DIRECTION ( 'NONE',  ( -1.000000000000000000, 0.000000000000000000, -0.000000000000000000 ) ) ;
#38064=DIRECTION ( 'NONE',  ( -0.000000000000000000, -0.000000000000000000, -1.000000000000000000 ) ) ;
#38071=LINE ( 'NONE', #9497, #48069 ) ;
#38077=ADVANCED_FACE ( 'NONE', ( #16162 ), #39099, .F. ) ;
#38078=FACE_OUTER_BOUND ( 'NONE', #34775, .T. ) ;
#38096=EDGE_CURVE ( 'NONE', #31369, #30416, #5651, .T. ) ;
#38115=ADVANCED_FACE ( 'NONE', ( #27811 ), #56773, .F. ) ;
#38121=CARTESIAN_POINT ( 'NONE',  ( -4.653126046682595884, -146.1313684676804314, -2.500000000000000000 ) ) ;
#38126=AXIS2_PLACEMENT_3D ( 'NONE', #58030, #53502, #47131 ) ;
#38134=LINE ( 'NONE', #72343, #32523 ) ;
#38153=EDGE_LOOP ( 'NONE', ( #66666, #69901, #39324, #57265 ) ) ;
#38265=DIRECTION ( 'NONE',  ( -0.9966891607226785466, -0.08130631524010122069, 0.000000000000000000 ) ) ;
#38286=CARTESIAN_POINT ( 'NONE',  ( -4.653126046682595884, -146.1313684676804314, 5.500000000000000000 ) ) ;
#38293=ADVANCED_FACE ( 'NONE', ( #48431 ), #53703, .F. ) ;
#38295=LINE ( 'NONE', #19239, #34070 ) ;
#38305=VERTEX_POINT ( 'NONE', #43560 ) ;
#38349=VECTOR ( 'NONE', #41630, 1000.000000000000227 ) ;
#38351=ORIENTED_EDGE ( 'NONE', *, *, #31815, .F. ) ;
#38387=EDGE_CURVE ( 'NONE', #43278, #39841, #42797, .T. ) ;
#38394=ORIENTED_EDGE ( 'NONE', *, *, #30619, .T. ) ;
#38411=VERTEX_POINT ( 'NONE', #49537 ) ;
#38413=VECTOR ( 'NONE', #5509, 1000.000000000000114 ) ;
#38432=ORIENTED_EDGE ( 'NONE', *, *, #15502, .F. ) ;
#38443=VECTOR ( 'NONE', #20996, 1000.000000000000000 ) ;
#38448=EDGE_LOOP ( 'NONE', ( #28734, #69445, #49837, #72772 ) ) ;
#38453=DIRECTION ( 'NONE',  ( -0.3853207896976547642, 0.9227826878668540234, 0.000000000000000000 ) ) ;
#38507=CYLINDRICAL_SURFACE ( 'NONE', #61263, 32.50000000000000000 ) ;
#38522=DIRECTION ( 'NONE',  ( -0.7585478161175723821, -0.6516173805718057377, 0.000000000000000000 ) ) ;
#38540=ORIENTED_EDGE ( 'NONE', *, *, #19522, .F. ) ;
#38563=VERTEX_POINT ( 'NONE', #7009 ) ;
#38564=VERTEX_POINT ( 'NONE', #58515 ) ;
#38580=ORIENTED_EDGE ( 'NONE', *, *, #29537, .T. ) ;
#38592=CARTESIAN_POINT ( 'NONE',  ( 8.700667342345820288, -98.11853780484867116, -5.500000000000000000 ) ) ;
#38599=LINE ( 'NONE', #58111, #53473 ) ;
#38600=CARTESIAN_POINT ( 'NONE',  ( 1.233757462863572574, -119.1468631277289347, 2.500000000000000000 ) ) ;
#38622=EDGE_CURVE ( 'NONE', #34951, #38411, #64173, .T. ) ;
#38623=FACE_OUTER_BOUND ( 'NONE', #52894, .T. ) ;
#38637=DIRECTION ( 'NONE',  ( -0.8090169943749426773, -0.5877852522924797984, 0.000000000000000000 ) ) ;
#38638=LINE ( 'NONE', #33733, #68212 ) ;
#38649=CARTESIAN_POINT ( 'NONE',  ( 22.94323693612312454, -114.6983135802921083, -2.500000000000000000 ) ) ;
#38654=EDGE_LOOP ( 'NONE', ( #44235, #31597, #7313, #20182 ) ) ;
#38657=VECTOR ( 'NONE', #14280, 1000.000000000000000 ) ;
#38684=DIRECTION ( 'NONE',  ( -0.02332147558787823344, -0.9997280174009349762, 0.000000000000000000 ) ) ;
#38688=ORIENTED_EDGE ( 'NONE', *, *, #49505, .F. ) ;
#38703=CARTESIAN_POINT ( 'NONE',  ( -25.50183398199384754, -112.6408924756582053, 5.500000000000000000 ) ) ;
#38707=CARTESIAN_POINT ( 'NONE',  ( -18.12185313557660038, -104.9634299478706794, -5.500000000000000000 ) ) ;
#38712=DIRECTION ( 'NONE',  ( -0.7585478161175716050, -0.6516173805718067369, 0.000000000000000000 ) ) ;
#38737=ORIENTED_EDGE ( 'NONE', *, *, #69944, .T. ) ;
#38745=ORIENTED_EDGE ( 'NONE', *, *, #42681, .F. ) ;
#38750=VERTEX_POINT ( 'NONE', #72008 ) ;
#38798=FACE_OUTER_BOUND ( 'NONE', #35033, .T. ) ;
#38801=VECTOR ( 'NONE', #16423, 1000.000000000000227 ) ;
#38804=DIRECTION ( 'NONE',  ( -0.9997280174009349762, 0.02332147558787671729, 0.000000000000000000 ) ) ;
#38810=EDGE_CURVE ( 'NONE', #52162, #44097, #3254, .T. ) ;
#38814=ORIENTED_EDGE ( 'NONE', *, *, #6612, .F. ) ;
#38826=VECTOR ( 'NONE', #23629, 1000.000000000000114 ) ;
#38863=DIRECTION ( 'NONE',  ( -0.000000000000000000, -0.000000000000000000, 1.000000000000000000 ) ) ;
#38871=ORIENTED_EDGE ( 'NONE', *, *, #51013, .F. ) ;
#38913=VERTEX_POINT ( 'NONE', #15621 ) ;
#38919=CIRCLE ( 'NONE', #70138, 35.50000000000000711 ) ;
#38930=CARTESIAN_POINT ( 'NONE',  ( 2.047646702416564768, -96.54137380445985173, 5.500000000000000000 ) ) ;
#38947=ORIENTED_EDGE ( 'NONE', *, *, #50023, .T. ) ;
#38948=CARTESIAN_POINT ( 'NONE',  ( 0.000000000000000000, -120.0000000000000000, -2.500000000000000000 ) ) ;
#38968=EDGE_CURVE ( 'NONE', #6231, #27626, #32527, .T. ) ;
#38992=FACE_OUTER_BOUND ( 'NONE', #40905, .T. ) ;
#39011=ORIENTED_EDGE ( 'NONE', *, *, #45332, .T. ) ;
#39045=PLANE ( 'NONE',  #52097 ) ;
#39059=EDGE_LOOP ( 'NONE', ( #71397, #24231, #53539, #70063 ) ) ;
#39069=VECTOR ( 'NONE', #35545, 1000.000000000000227 ) ;
#39073=FACE_OUTER_BOUND ( 'NONE', #11406, .T. ) ;
#39077=ADVANCED_FACE ( 'NONE', ( #54448 ), #8208, .F. ) ;
#39079=DIRECTION ( 'NONE',  ( 0.7950889364178798102, -0.6064928550163511956, 0.000000000000000000 ) ) ;
#39093=FACE_OUTER_BOUND ( 'NONE', #6341, .T. ) ;
#39099=PLANE ( 'NONE',  #30767 ) ;
#39109=EDGE_LOOP ( 'NONE', ( #41991, #71617, #20338, #22369 ) ) ;
#39115=FACE_OUTER_BOUND ( 'NONE', #10081, .T. ) ;
#39126=VERTEX_POINT ( 'NONE', #38649 ) ;
#39158=VECTOR ( 'NONE', #56565, 1000.000000000000114 ) ;
#39182=LINE ( 'NONE', #55354, #46188 ) ;
#39198=CARTESIAN_POINT ( 'NONE',  ( 22.08297821871651934, -111.8242998470044540, 5.500000000000000000 ) ) ;
#39200=PLANE ( 'NONE',  #57490 ) ;
#39216=CARTESIAN_POINT ( 'NONE',  ( 8.700667342345820288, -98.11853780484867116, 2.500000000000000000 ) ) ;
#39264=FACE_OUTER_BOUND ( 'NONE', #54118, .T. ) ;
#39277=DIRECTION ( 'NONE',  ( -0.000000000000000000, -0.000000000000000000, -1.000000000000000000 ) ) ;
#39297=EDGE_CURVE ( 'NONE', #41422, #6148, #13020, .T. ) ;
#39302=CARTESIAN_POINT ( 'NONE',  ( -30.50000000000000000, -120.0000000000000000, -5.500000000000000000 ) ) ;
#39322=ORIENTED_EDGE ( 'NONE', *, *, #49410, .F. ) ;
#39324=ORIENTED_EDGE ( 'NONE', *, *, #46250, .F. ) ;
#39337=EDGE_CURVE ( 'NONE', #9704, #30416, #23571, .T. ) ;
#39356=DIRECTION ( 'NONE',  ( 1.000000000000000000, 0.000000000000000000, 0.000000000000000000 ) ) ;
#39380=VECTOR ( 'NONE', #55847, 1000.000000000000000 ) ;
#39381=EDGE_CURVE ( 'NONE', #56786, #1038, #64602, .T. ) ;
#39384=ORIENTED_EDGE ( 'NONE', *, *, #1253, .F. ) ;
#39417=VECTOR ( 'NONE', #68682, 1000.000000000000000 ) ;
#39418=CARTESIAN_POINT ( 'NONE',  ( -13.05994868825747446, -139.5943292883446532, 5.500000000000000000 ) ) ;
#39422=LINE ( 'NONE', #20998, #45324 ) ;
#39450=DIRECTION ( 'NONE',  ( -0.4279312458752990711, -0.9038112904824846527, 0.000000000000000000 ) ) ;
#39454=PLANE ( 'NONE',  #3892 ) ;
#39455=AXIS2_PLACEMENT_3D ( 'NONE', #18101, #41760, #63611 ) ;
#39461=CARTESIAN_POINT ( 'NONE',  ( -3.961125083139900749, -143.2122702051246677, -5.500000000000000000 ) ) ;
#39465=DIRECTION ( 'NONE',  ( -0.8774505977381983346, -0.4796670183876294291, 0.000000000000000000 ) ) ;
#39480=CARTESIAN_POINT ( 'NONE',  ( 103.9230484541331947, -179.9999999999990337, -5.500000000000000000 ) ) ;
#39496=CARTESIAN_POINT ( 'NONE',  ( 12.50000000000000000, -107.5000000000000000, 2.500000000000000000 ) ) ;
#39537=ORIENTED_EDGE ( 'NONE', *, *, #32557, .F. ) ;
#39538=VECTOR ( 'NONE', #3677, 1000.000000000000000 ) ;
#39553=DIRECTION ( 'NONE',  ( -0.000000000000000000, -0.000000000000000000, 1.000000000000000000 ) ) ;
#39560=ORIENTED_EDGE ( 'NONE', *, *, #61277, .F. ) ;
#39569=VECTOR ( 'NONE', #19469, 1000.000000000000114 ) ;
#39576=EDGE_LOOP ( 'NONE', ( #36318, #21835, #24364, #66760 ) ) ;
#39599=CARTESIAN_POINT ( 'NONE',  ( -25.50183398199384754, -112.6408924756582053, 5.500000000000000000 ) ) ;
#39628=ADVANCED_FACE ( 'NONE', ( #41067 ), #10349, .F. ) ;
#39663=ADVANCED_FACE ( 'NONE', ( #73122 ), #45322, .F. ) ;
#39665=DIRECTION ( 'NONE',  ( 0.4796670183876317051, -0.8774505977381972244, 0.000000000000000000 ) ) ;
#39675=EDGE_CURVE ( 'NONE', #40375, #22108, #50186, .T. ) ;
#39683=EDGE_CURVE ( 'NONE', #30034, #71014, #50567, .T. ) ;
#39694=DIRECTION ( 'NONE',  ( -0.9730327541852497042, 0.2306669878475623159, 0.000000000000000000 ) ) ;
#39709=AXIS2_PLACEMENT_3D ( 'NONE', #37681, #4218, #62093 ) ;
#39766=DIRECTION ( 'NONE',  ( 1.000000000000000000, 0.000000000000000000, 0.000000000000000000 ) ) ;
#39790=DIRECTION ( 'NONE',  ( -0.6516173805718079581, 0.7585478161175704948, 0.000000000000000000 ) ) ;
#39793=CIRCLE ( 'NONE', #45816, 32.50000000000000000 ) ;
#39815=VECTOR ( 'NONE', #18516, 1000.000000000000114 ) ;
#39825=CARTESIAN_POINT ( 'NONE',  ( 5.822613034544236399, -142.8165987265839476, -2.500000000000000000 ) ) ;
#39841=VERTEX_POINT ( 'NONE', #24151 ) ;
#39854=DIRECTION ( 'NONE',  ( 0.4796670183876317051, -0.8774505977381971134, 0.000000000000000000 ) ) ;
#39855=EDGE_LOOP ( 'NONE', ( #24671, #44064, #6347, #25809 ) ) ;
#39883=ORIENTED_EDGE ( 'NONE', *, *, #10595, .T. ) ;
#39905=DIRECTION ( 'NONE',  ( -0.4796670183876317051, 0.8774505977381971134, 0.000000000000000000 ) ) ;
#39937=CARTESIAN_POINT ( 'NONE',  ( -24.50849501662245800, -109.8101191361138831, 5.500000000000000000 ) ) ;
#39959=ORIENTED_EDGE ( 'NONE', *, *, #8576, .F. ) ;
#39983=LINE ( 'NONE', #58372, #47621 ) ;
#39994=LINE ( 'NONE', #50890, #6692 ) ;
#40004=LINE ( 'NONE', #35100, #60789 ) ;
#40046=LINE ( 'NONE', #45706, #58671 ) ;
#40052=CARTESIAN_POINT ( 'NONE',  ( -19.90058851926621131, -132.5883508287165853, 5.500000000000000000 ) ) ;
#40066=DIRECTION ( 'NONE',  ( -0.9827303690289279636, -0.1850432970638682117, 0.000000000000000000 ) ) ;
#40074=CARTESIAN_POINT ( 'NONE',  ( 26.47460221209471598, -121.8961639463267090, 5.500000000000000000 ) ) ;
#40087=EDGE_CURVE ( 'NONE', #37730, #68048, #34216, .T. ) ;
#40091=DIRECTION ( 'NONE',  ( 0.2306669878475623159, 0.9730327541852497042, -0.000000000000000000 ) ) ;
#40106=ORIENTED_EDGE ( 'NONE', *, *, #36903, .F. ) ;
#40112=AXIS2_PLACEMENT_3D ( 'NONE', #64273, #12748, #64633 ) ;
#40148=AXIS2_PLACEMENT_3D ( 'NONE', #28047, #74287, #11497 ) ;
#40151=EDGE_CURVE ( 'NONE', #20908, #31608, #68444, .T. ) ;
#40155=CARTESIAN_POINT ( 'NONE',  ( 17.82587367876289974, -104.6869915565625320, 2.500000000000000000 ) ) ;
#40158=EDGE_CURVE ( 'NONE', #1173, #12862, #34582, .T. ) ;
#40173=ORIENTED_EDGE ( 'NONE', *, *, #30825, .F. ) ;
#40215=EDGE_LOOP ( 'NONE', ( #41420, #19584, #56099, #68142 ) ) ;
#40218=ORIENTED_EDGE ( 'NONE', *, *, #883, .F. ) ;
#40232=DIRECTION ( 'NONE',  ( -0.000000000000000000, -0.000000000000000000, -1.000000000000000000 ) ) ;
#40287=DIRECTION ( 'NONE',  ( 1.000000000000000000, 0.000000000000000000, 0.000000000000000000 ) ) ;
#40292=VECTOR ( 'NONE', #15884, 1000.000000000000114 ) ;
#40306=VERTEX_POINT ( 'NONE', #7860 ) ;
#40311=ORIENTED_EDGE ( 'NONE', *, *, #46443, .T. ) ;
#40320=VERTEX_POINT ( 'NONE', #24412 ) ;
#40323=VERTEX_POINT ( 'NONE', #18039 ) ;
#40339=ORIENTED_EDGE ( 'NONE', *, *, #2957, .T. ) ;
#40346=CARTESIAN_POINT ( 'NONE',  ( 24.95699195200416654, -110.9640411295978595, 5.500000000000000000 ) ) ;
#40360=LINE ( 'NONE', #13536, #11147 ) ;
#40362=LINE ( 'NONE', #58389, #51649 ) ;
#40375=VERTEX_POINT ( 'NONE', #2639 ) ;
#40377=CARTESIAN_POINT ( 'NONE',  ( -4.653126046682595884, -146.1313684676804314, -5.500000000000000000 ) ) ;
#40394=VECTOR ( 'NONE', #37537, 1000.000000000000114 ) ;
#40398=CARTESIAN_POINT ( 'NONE',  ( -15.44521549751111422, -137.7748507232956001, 5.500000000000000000 ) ) ;
#40406=VERTEX_POINT ( 'NONE', #55947 ) ;
#40419=EDGE_CURVE ( 'NONE', #3158, #21881, #8972, .T. ) ;
#40441=AXIS2_PLACEMENT_3D ( 'NONE', #50619, #73546, #45752 ) ;
#40446=FACE_OUTER_BOUND ( 'NONE', #3476, .T. ) ;
#40452=LINE ( 'NONE', #22812, #39069 ) ;
#40458=DIRECTION ( 'NONE',  ( 0.2867529058022035837, -0.9580045777625452175, 0.000000000000000000 ) ) ;
#40462=CARTESIAN_POINT ( 'NONE',  ( 0.1915406271734537980, -118.5122795329289858, 2.500000000000000000 ) ) ;
#40486=VERTEX_POINT ( 'NONE', #71736 ) ;
#40492=CARTESIAN_POINT ( 'NONE',  ( 5.822613034544236399, -142.8165987265839760, 2.500000000000000000 ) ) ;
#40511=EDGE_CURVE ( 'NONE', #47167, #40375, #26626, .T. ) ;
#40557=LINE ( 'NONE', #384, #20536 ) ;
#40588=VECTOR ( 'NONE', #19730, 1000.000000000000000 ) ;
#40591=CARTESIAN_POINT ( 'NONE',  ( 18.80329974962065265, -105.8248132807389084, 5.500000000000000000 ) ) ;
#40621=VECTOR ( 'NONE', #65930, 1000.000000000000000 ) ;
#40648=EDGE_CURVE ( 'NONE', #72033, #51387, #69091, .T. ) ;
#40665=DIRECTION ( 'NONE',  ( 0.000000000000000000, 0.000000000000000000, 1.000000000000000000 ) ) ;
#40696=VECTOR ( 'NONE', #41159, 1000.000000000000000 ) ;
#40709=DIRECTION ( 'NONE',  ( 1.000000000000000000, 0.000000000000000000, 0.000000000000000000 ) ) ;
#40725=LINE ( 'NONE', #30531, #48705 ) ;
#40750=DIRECTION ( 'NONE',  ( -0.000000000000000000, -0.000000000000000000, -1.000000000000000000 ) ) ;
#40770=EDGE_CURVE ( 'NONE', #35029, #14025, #1092, .T. ) ;
#40794=VERTEX_POINT ( 'NONE', #13787 ) ;
#40795=LINE ( 'NONE', #11104, #56311 ) ;
#40803=DIRECTION ( 'NONE',  ( 0.8541291221503265474, -0.5200609990133007177, 0.000000000000000000 ) ) ;
#40826=EDGE_CURVE ( 'NONE', #58064, #9787, #58549, .T. ) ;
#40845=DIRECTION ( 'NONE',  ( 0.6516173805718058487, -0.7585478161175724932, 0.000000000000000000 ) ) ;
#40878=VECTOR ( 'NONE', #16783, 1000.000000000000000 ) ;
#40880=EDGE_LOOP ( 'NONE', ( #54850, #1040, #49179, #16868 ) ) ;
#40887=DIRECTION ( 'NONE',  ( -0.7273375899149793211, 0.6862798483830554463, 0.000000000000000000 ) ) ;
#40905=EDGE_LOOP ( 'NONE', ( #50218, #55973, #47534, #55884 ) ) ;
#40920=CARTESIAN_POINT ( 'NONE',  ( -16.06301359042743115, -102.7814171781257357, -5.500000000000000000 ) ) ;
#40924=EDGE_LOOP ( 'NONE', ( #13500, #24771, #170, #32519 ) ) ;
#40926=DIRECTION ( 'NONE',  ( 0.6516173805718078471, -0.7585478161175706058, 0.000000000000000000 ) ) ;
#40952=DIRECTION ( 'NONE',  ( -0.000000000000000000, -0.000000000000000000, 1.000000000000000000 ) ) ;
#41012=EDGE_CURVE ( 'NONE', #72033, #48661, #16778, .T. ) ;
#41027=AXIS2_PLACEMENT_3D ( 'NONE', #26734, #26372, #16580 ) ;
#41040=ORIENTED_EDGE ( 'NONE', *, *, #43558, .F. ) ;
#41046=DIRECTION ( 'NONE',  ( 1.000000000000000000, 0.000000000000000000, -0.000000000000000000 ) ) ;
#41063=LINE ( 'NONE', #28375, #10097 ) ;
#41067=FACE_OUTER_BOUND ( 'NONE', #46889, .T. ) ;
#41100=CARTESIAN_POINT ( 'NONE',  ( 30.50000000000000000, -120.0000000000000000, 2.500000000000000000 ) ) ;
#41105=ORIENTED_EDGE ( 'NONE', *, *, #28414, .T. ) ;
#41124=( NAMED_UNIT ( * ) PLANE_ANGLE_UNIT ( ) SI_UNIT ( $, .RADIAN. ) );
#41133=DIRECTION ( 'NONE',  ( -0.000000000000000000, -0.000000000000000000, -1.000000000000000000 ) ) ;
#41147=ORIENTED_EDGE ( 'NONE', *, *, #26838, .F. ) ;
#41159=DIRECTION ( 'NONE',  ( -0.000000000000000000, -0.000000000000000000, -1.000000000000000000 ) ) ;
#41163=EDGE_CURVE ( 'NONE', #41422, #45134, #16397, .T. ) ;
#41169=ADVANCED_FACE ( 'NONE', ( #73528 ), #68657, .F. ) ;
#41187=EDGE_LOOP ( 'NONE', ( #54244, #48329, #36604, #9525 ) ) ;
#41192=DIRECTION ( 'NONE',  ( -0.8774505977381978905, -0.4796670183876304283, 0.000000000000000000 ) ) ;
#41222=CARTESIAN_POINT ( 'NONE',  ( 16.84844760790522145, -103.5491698323862124, -2.500000000000000000 ) ) ;
#41223=CARTESIAN_POINT ( 'NONE',  ( 0.000000000000000000, -120.0000000000000000, 2.500000000000000000 ) ) ;
#41279=DIRECTION ( 'NONE',  ( 0.9038112904824842087, -0.4279312458753000703, 0.000000000000000000 ) ) ;
#41297=CARTESIAN_POINT ( 'NONE',  ( -6.880223345695647197, -142.5202692415819854, 5.500000000000000000 ) ) ;
#41324=ORIENTED_EDGE ( 'NONE', *, *, #50351, .T. ) ;
#41333=FACE_OUTER_BOUND ( 'NONE', #39855, .T. ) ;
#41351=CARTESIAN_POINT ( 'NONE',  ( -18.24502636017238899, -100.7225776329765665, 5.500000000000000000 ) ) ;
#41365=DIRECTION ( 'NONE',  ( -0.1850432970638656582, 0.9827303690289285187, 0.000000000000000000 ) ) ;
#41390=LINE ( 'NONE', #1219, #4018 ) ;
#41395=CARTESIAN_POINT ( 'NONE',  ( 14.59956846177685996, -138.4757300459248484, 5.500000000000000000 ) ) ;
#41399=CARTESIAN_POINT ( 'NONE',  ( 89.17737905728634473, -39.70432723693593857, -5.500000000000000000 ) ) ;
#41405=CARTESIAN_POINT ( 'NONE',  ( 21.85433023846371370, -135.0628101570779620, -5.500000000000000000 ) ) ;
#41407=SURFACE_STYLE_FILL_AREA ( #13562 ) ;
#41417=ORIENTED_EDGE ( 'NONE', *, *, #55919, .F. ) ;
#41420=ORIENTED_EDGE ( 'NONE', *, *, #54477, .F. ) ;
#41422=VERTEX_POINT ( 'NONE', #3938 ) ;
#41427=EDGE_CURVE ( 'NONE', #17454, #45219, #3571, .T. ) ;
#41454=CARTESIAN_POINT ( 'NONE',  ( -3.961125083139900749, -143.2122702051246677, 5.500000000000000000 ) ) ;
#41508=VERTEX_POINT ( 'NONE', #56549 ) ;
#41510=ORIENTED_EDGE ( 'NONE', *, *, #1266, .F. ) ;
#41515=DIRECTION ( 'NONE',  ( -0.000000000000000000, -0.000000000000000000, -1.000000000000000000 ) ) ;
#41542=DIRECTION ( 'NONE',  ( 0.02332147558787931590, 0.9997280174009348652, 0.000000000000000000 ) ) ;
#41543=DIRECTION ( 'NONE',  ( 0.9227826878668540234, 0.3853207896976547087, 0.000000000000000000 ) ) ;
#41561=CARTESIAN_POINT ( 'NONE',  ( 21.07894319797337346, -103.8699611390234878, 2.500000000000000000 ) ) ;
#41581=EDGE_CURVE ( 'NONE', #11006, #47167, #50125, .T. ) ;
#41595=DIRECTION ( 'NONE',  ( -0.000000000000000000, -0.000000000000000000, -1.000000000000000000 ) ) ;
#41630=DIRECTION ( 'NONE',  ( 0.9580045777625458836, 0.2867529058022011412, -0.000000000000000000 ) ) ;
#41640=ORIENTED_EDGE ( 'NONE', *, *, #22990, .T. ) ;
#41642=CARTESIAN_POINT ( 'NONE',  ( 22.08297821871651934, -111.8242998470044540, -5.500000000000000000 ) ) ;
#41660=CARTESIAN_POINT ( 'NONE',  ( 0.000000000000000000, -120.0000000000000000, 2.500000000000000000 ) ) ;
#41666=LINE ( 'NONE', #46575, #28876 ) ;
#41670=DIRECTION ( 'NONE',  ( 0.000000000000000000, 0.000000000000000000, 1.000000000000000000 ) ) ;
#41672=VECTOR ( 'NONE', #52209, 1000.000000000000000 ) ;
#41688=LINE ( 'NONE', #54096, #56351 ) ;
#41696=DIRECTION ( 'NONE',  ( -0.000000000000000000, -0.000000000000000000, 1.000000000000000000 ) ) ;
#41712=FACE_BOUND ( 'NONE', #42190, .T. ) ;
#41723=ORIENTED_EDGE ( 'NONE', *, *, #45950, .F. ) ;
#41726=ORIENTED_EDGE ( 'NONE', *, *, #24111, .F. ) ;
#41753=FACE_OUTER_BOUND ( 'NONE', #70719, .T. ) ;
#41760=DIRECTION ( 'NONE',  ( 0.6064928550163511956, 0.7950889364178798102, -0.000000000000000000 ) ) ;
#41770=FILL_AREA_STYLE_COLOUR ( '', #61989 ) ;
#41771=ORIENTED_EDGE ( 'NONE', *, *, #69511, .F. ) ;
#41778=FACE_BOUND ( 'NONE', #22322, .T. ) ;
#41781=VECTOR ( 'NONE', #58905, 1000.000000000000114 ) ;
#41785=LINE ( 'NONE', #2351, #22077 ) ;
#41820=VECTOR ( 'NONE', #73828, 1000.000000000000000 ) ;
#41841=EDGE_CURVE ( 'NONE', #52067, #33176, #71493, .T. ) ;
#41850=AXIS2_PLACEMENT_3D ( 'NONE', #54542, #8686, #65829 ) ;
#41889=EDGE_LOOP ( 'NONE', ( #33101, #66835, #49719, #27290 ) ) ;
#41926=EDGE_CURVE ( 'NONE', #45726, #68048, #32382, .T. ) ;
#41940=DIRECTION ( 'NONE',  ( -0.9827303690289279636, -0.1850432970638682117, 0.000000000000000000 ) ) ;
#41951=EDGE_CURVE ( 'NONE', #8033, #54914, #49309, .T. ) ;
#41988=ORIENTED_EDGE ( 'NONE', *, *, #25204, .F. ) ;
#41991=ORIENTED_EDGE ( 'NONE', *, *, #42515, .F. ) ;
#41994=DIRECTION ( 'NONE',  ( -0.000000000000000000, -0.000000000000000000, 1.000000000000000000 ) ) ;
#42017=ORIENTED_EDGE ( 'NONE', *, *, #28330, .T. ) ;
#42027=ORIENTED_EDGE ( 'NONE', *, *, #59169, .F. ) ;
#42051=FACE_OUTER_BOUND ( 'NONE', #27450, .T. ) ;
#42053=DIRECTION ( 'NONE',  ( 0.8225049752423776450, 0.5687579148473765889, -0.000000000000000000 ) ) ;
#42061=AXIS2_PLACEMENT_3D ( 'NONE', #56666, #6900, #28064 ) ;
#42132=EDGE_CURVE ( 'NONE', #19022, #9704, #4793, .T. ) ;
#42142=DIRECTION ( 'NONE',  ( 0.000000000000000000, -0.000000000000000000, -1.000000000000000000 ) ) ;
#42171=VERTEX_POINT ( 'NONE', #26574 ) ;
#42181=ORIENTED_EDGE ( 'NONE', *, *, #3592, .F. ) ;
#42185=VERTEX_POINT ( 'NONE', #52100 ) ;
#42190=EDGE_LOOP ( 'NONE', ( #72187, #1231, #50741, #50558 ) ) ;
#42204=EDGE_CURVE ( 'NONE', #31960, #9134, #57380, .T. ) ;
#42212=AXIS2_PLACEMENT_3D ( 'NONE', #67272, #26662, #15765 ) ;
#42224=LINE ( 'NONE', #60258, #58614 ) ;
#42245=DIRECTION ( 'NONE',  ( -0.000000000000000000, -0.000000000000000000, -1.000000000000000000 ) ) ;
#42249=ADVANCED_FACE ( 'NONE', ( #23533 ), #29160, .F. ) ;
#42256=( GEOMETRIC_REPRESENTATION_CONTEXT ( 3 ) GLOBAL_UNCERTAINTY_ASSIGNED_CONTEXT ( ( #9168 ) ) GLOBAL_UNIT_ASSIGNED_CONTEXT ( ( #64422, #35826, #64794 ) ) REPRESENTATION_CONTEXT ( 'NONE', 'WORKASPACE' ) );
#42274=EDGE_CURVE ( 'NONE', #25489, #72033, #40452, .T. ) ;
#42276=ADVANCED_FACE ( 'NONE', ( #17887 ), #23176, .F. ) ;
#42288=CARTESIAN_POINT ( 'NONE',  ( -14.87942725330654348, -141.9795960975983178, 2.500000000000000000 ) ) ;
#42293=ORIENTED_EDGE ( 'NONE', *, *, #42204, .F. ) ;
#42307=CARTESIAN_POINT ( 'NONE',  ( 26.09152095774781799, -124.8716048804687375, -5.500000000000000000 ) ) ;
#42319=LINE ( 'NONE', #65253, #68949 ) ;
#42334=VECTOR ( 'NONE', #46646, 1000.000000000000114 ) ;
#42348=LINE ( 'NONE', #2541, #26779 ) ;
#42353=ORIENTED_EDGE ( 'NONE', *, *, #44555, .F. ) ;
#42365=ORIENTED_EDGE ( 'NONE', *, *, #67900, .F. ) ;
#42374=EDGE_CURVE ( 'NONE', #27626, #69665, #25006, .T. ) ;
#42376=CARTESIAN_POINT ( 'NONE',  ( -16.06301359042743115, -102.7814171781257357, 5.500000000000000000 ) ) ;
#42378=PLANE ( 'NONE',  #5939 ) ;
#42393=VERTEX_POINT ( 'NONE', #53219 ) ;
#42399=DIRECTION ( 'NONE',  ( -0.9918136447140101231, 0.1276937514489694114, 0.000000000000000000 ) ) ;
#42403=CARTESIAN_POINT ( 'NONE',  ( -1.474095553543409487, -120.2775649455957989, 2.500000000000000000 ) ) ;
#42415=ORIENTED_EDGE ( 'NONE', *, *, #21102, .F. ) ;
#42425=AXIS2_PLACEMENT_3D ( 'NONE', #22818, #57023, #46109 ) ;
#42436=CARTESIAN_POINT ( 'NONE',  ( 12.50000000000000000, -107.5000000000000000, -2.500000000000000000 ) ) ;
#42444=CARTESIAN_POINT ( 'NONE',  ( 3.429551818649054340, -146.3199197248623875, 5.500000000000000000 ) ) ;
#42454=VERTEX_POINT ( 'NONE', #20099 ) ;
#42464=PLANE ( 'NONE',  #29669 ) ;
#42479=ORIENTED_EDGE ( 'NONE', *, *, #55536, .T. ) ;
#42483=DIRECTION ( 'NONE',  ( 0.3853207896976533209, -0.9227826878668545785, 0.000000000000000000 ) ) ;
#42515=EDGE_CURVE ( 'NONE', #56886, #22041, #33229, .T. ) ;
#42526=FACE_BOUND ( 'NONE', #59253, .T. ) ;
#42564=PLANE ( 'NONE',  #10689 ) ;
#42603=LINE ( 'NONE', #61377, #47804 ) ;
#42614=CARTESIAN_POINT ( 'NONE',  ( -23.54415474984308787, -120.4156646670583086, 5.500000000000000000 ) ) ;
#42659=DIRECTION ( 'NONE',  ( -0.9781476007338069101, 0.2079116908177532363, 0.000000000000000000 ) ) ;
#42678=DIRECTION ( 'NONE',  ( -0.2306669878475622604, -0.9730327541852497042, 0.000000000000000000 ) ) ;
#42681=EDGE_CURVE ( 'NONE', #43075, #55006, #60705, .T. ) ;
#42723=EDGE_LOOP ( 'NONE', ( #58799, #72028, #63090, #12402 ) ) ;
#42724=LINE ( 'NONE', #30683, #29781 ) ;
#42731=VERTEX_POINT ( 'NONE', #51652 ) ;
#42750=ORIENTED_EDGE ( 'NONE', *, *, #56006, .T. ) ;
#42767=DIRECTION ( 'NONE',  ( -0.08130631524010117905, 0.9966891607226784355, 0.000000000000000000 ) ) ;
#42780=ORIENTED_EDGE ( 'NONE', *, *, #41581, .T. ) ;
#42782=DIRECTION ( 'NONE',  ( 0.5200609990132993854, 0.8541291221503275466, 0.000000000000000000 ) ) ;
#42797=LINE ( 'NONE', #26604, #40394 ) ;
#42802=AXIS2_PLACEMENT_3D ( 'NONE', #3386, #49221, #15008 ) ;
#42811=DIRECTION ( 'NONE',  ( 0.3311129884571281101, 0.9435911131814402886, -0.000000000000000000 ) ) ;
#42832=VECTOR ( 'NONE', #50051, 1000.000000000000114 ) ;
#42850=CARTESIAN_POINT ( 'NONE',  ( 11.41210121379328335, -99.40233154247455616, 5.500000000000000000 ) ) ;
#42922=DIRECTION ( 'NONE',  ( 0.3853207896976533209, -0.9227826878668545785, 0.000000000000000000 ) ) ;
#42924=ORIENTED_EDGE ( 'NONE', *, *, #69620, .F. ) ;
#42940=DIRECTION ( 'NONE',  ( 0.9966891607226785466, 0.08130631524009969413, 0.000000000000000000 ) ) ;
#42977=DIRECTION ( 'NONE',  ( -0.8774505977381983346, -0.4796670183876294291, 0.000000000000000000 ) ) ;
#42983=EDGE_CURVE ( 'NONE', #59758, #45592, #12966, .T. ) ;
#42984=AXIS2_PLACEMENT_3D ( 'NONE', #38930, #56603, #50945 ) ;
#42996=ORIENTED_EDGE ( 'NONE', *, *, #59021, .T. ) ;
#42997=ORIENTED_EDGE ( 'NONE', *, *, #47393, .F. ) ;
#43002=ORIENTED_EDGE ( 'NONE', *, *, #59816, .F. ) ;
#43006=CARTESIAN_POINT ( 'NONE',  ( -12.50000000000000000, -107.5000000000000000, -2.500000000000000000 ) ) ;
#43051=LINE ( 'NONE', #25000, #72307 ) ;
#43072=VECTOR ( 'NONE', #18996, 1000.000000000000000 ) ;
#43075=VERTEX_POINT ( 'NONE', #26399 ) ;
#43088=VECTOR ( 'NONE', #38522, 1000.000000000000114 ) ;
#43093=DIRECTION ( 'NONE',  ( -0.7585478161175706058, -0.6516173805718078471, 0.000000000000000000 ) ) ;
#43129=LINE ( 'NONE', #49850, #10225 ) ;
#43130=DIRECTION ( 'NONE',  ( 0.000000000000000000, -0.000000000000000000, 1.000000000000000000 ) ) ;
#43152=LINE ( 'NONE', #2944, #59944 ) ;
#43173=CARTESIAN_POINT ( 'NONE',  ( 21.07894319797337701, -103.8699611390234878, -2.500000000000000444 ) ) ;
#43183=AXIS2_PLACEMENT_3D ( 'NONE', #22455, #15698, #38637 ) ;
#43186=EDGE_CURVE ( 'NONE', #43075, #42393, #71509, .T. ) ;
#43204=ORIENTED_EDGE ( 'NONE', *, *, #44555, .T. ) ;
#43216=ORIENTED_EDGE ( 'NONE', *, *, #3870, .F. ) ;
#43218=EDGE_CURVE ( 'NONE', #7502, #52797, #62102, .T. ) ;
#43243=CIRCLE ( 'NONE', #54009, 30.50000000000000000 ) ;
#43245=CARTESIAN_POINT ( 'NONE',  ( -17.26469406256017791, -140.1601175325492648, 5.500000000000000000 ) ) ;
#43269=EDGE_LOOP ( 'NONE', ( #46707, #268, #16309, #44203 ) ) ;
#43278=VERTEX_POINT ( 'NONE', #21870 ) ;
#43287=VECTOR ( 'NONE', #57021, 1000.000000000000000 ) ;
#43290=ORIENTED_EDGE ( 'NONE', *, *, #73766, .T. ) ;
#43308=PLANE ( 'NONE',  #28063 ) ;
#43343=LINE ( 'NONE', #8741, #26575 ) ;
#43347=AXIS2_PLACEMENT_3D ( 'NONE', #12980, #40845, #70126 ) ;
#43361=VERTEX_POINT ( 'NONE', #24830 ) ;
#43372=ORIENTED_EDGE ( 'NONE', *, *, #4776, .F. ) ;
#43389=EDGE_CURVE ( 'NONE', #30416, #46309, #70674, .T. ) ;
#43395=AXIS2_PLACEMENT_3D ( 'NONE', #48320, #71232, #19735 ) ;
#43396=VECTOR ( 'NONE', #17500, 1000.000000000000000 ) ;
#43397=ORIENTED_EDGE ( 'NONE', *, *, #37848, .F. ) ;
#43453=VERTEX_POINT ( 'NONE', #2315 ) ;
#43477=LINE ( 'NONE', #31782, #64060 ) ;
#43496=ORIENTED_EDGE ( 'NONE', *, *, #36815, .T. ) ;
#43504=LINE ( 'NONE', #3649, #69420 ) ;
#43512=ADVANCED_FACE ( 'NONE', ( #52294 ), #837, .F. ) ;
#43558=EDGE_CURVE ( 'NONE', #38750, #61799, #16803, .T. ) ;
#43560=CARTESIAN_POINT ( 'NONE',  ( 2.047646702416564768, -96.54137380445985173, -5.500000000000000000 ) ) ;
#43572=VECTOR ( 'NONE', #69577, 1000.000000000000000 ) ;
#43573=CARTESIAN_POINT ( 'NONE',  ( 19.12409105625795291, -101.5943176906707919, 5.500000000000000000 ) ) ;
#43574=ORIENTED_EDGE ( 'NONE', *, *, #20173, .F. ) ;
#43584=DIRECTION ( 'NONE',  ( 0.9038112904824853189, -0.4279312458752977388, 0.000000000000000000 ) ) ;
#43595=ORIENTED_EDGE ( 'NONE', *, *, #46443, .F. ) ;
#43605=PLANE ( 'NONE',  #60927 ) ;
#43616=CARTESIAN_POINT ( 'NONE',  ( -13.05994868825747446, -139.5943292883446532, 2.500000000000000000 ) ) ;
#43623=VECTOR ( 'NONE', #56747, 1000.000000000000114 ) ;
#43624=DIRECTION ( 'NONE',  ( -0.9997280174009349762, 0.02332147558787674504, 0.000000000000000000 ) ) ;
#43628=ADVANCED_FACE ( 'NONE', ( #3045 ), #20297, .F. ) ;
#43631=VERTEX_POINT ( 'NONE', #28065 ) ;
#43648=ORIENTED_EDGE ( 'NONE', *, *, #72485, .F. ) ;
#43654=ORIENTED_EDGE ( 'NONE', *, *, #60061, .F. ) ;
#43655=PLANE ( 'NONE',  #1676 ) ;
#43669=VERTEX_POINT ( 'NONE', #2043 ) ;
#43701=CARTESIAN_POINT ( 'NONE',  ( -17.09243336300205129, -103.8724235629982502, -2.500000000000000000 ) ) ;
#43723=CARTESIAN_POINT ( 'NONE',  ( 2.047646702416564768, -96.54137380445985173, -5.500000000000000000 ) ) ;
#43730=CARTESIAN_POINT ( 'NONE',  ( 23.49916127795269460, -121.5130826919798039, -5.500000000000000000 ) ) ;
#43738=PLANE ( 'NONE',  #66669 ) ;
#43742=VERTEX_POINT ( 'NONE', #2784 ) ;
#43750=ORIENTED_EDGE ( 'NONE', *, *, #55019, .F. ) ;
#43777=VECTOR ( 'NONE', #38064, 1000.000000000000000 ) ;
#43778=CARTESIAN_POINT ( 'NONE',  ( 19.29194287201271862, -133.5026271600380880, -5.500000000000000000 ) ) ;
#43779=DIRECTION ( 'NONE',  ( -0.000000000000000000, -0.000000000000000000, -1.000000000000000000 ) ) ;
#43789=CIRCLE ( 'NONE', #11340, 35.50000000000000711 ) ;
#43815=ORIENTED_EDGE ( 'NONE', *, *, #54519, .T. ) ;
#43824=DIRECTION ( 'NONE',  ( 0.08130631524010117905, -0.9966891607226784355, 0.000000000000000000 ) ) ;
#43835=CARTESIAN_POINT ( 'NONE',  ( 1.474095553543393056, -119.7224350544041869, -2.500000000000000000 ) ) ;
#43857=DIRECTION ( 'NONE',  ( 0.7585478161175723821, 0.6516173805718057377, -0.000000000000000000 ) ) ;
#43862=DIRECTION ( 'NONE',  ( -0.000000000000000000, -0.000000000000000000, -1.000000000000000000 ) ) ;
#43867=ORIENTED_EDGE ( 'NONE', *, *, #28203, .F. ) ;
#43877=ORIENTED_EDGE ( 'NONE', *, *, #12745, .F. ) ;
#43883=DIRECTION ( 'NONE',  ( 0.000000000000000000, 0.000000000000000000, 1.000000000000000000 ) ) ;
#43889=PLANE ( 'NONE',  #71270 ) ;
#43907=CARTESIAN_POINT ( 'NONE',  ( 6.377742925735834234, -145.7647898336708181, 5.500000000000000000 ) ) ;
#43914=ADVANCED_FACE ( 'NONE', ( #22629 ), #12081, .F. ) ;
#43930=FACE_OUTER_BOUND ( 'NONE', #65744, .T. ) ;
#43933=AXIS2_PLACEMENT_3D ( 'NONE', #46755, #195, #17437 ) ;
#43949=ORIENTED_EDGE ( 'NONE', *, *, #45332, .F. ) ;
#43950=DIRECTION ( 'NONE',  ( -0.9997280174009349762, 0.02332147558787823691, 0.000000000000000000 ) ) ;
#43972=DIRECTION ( 'NONE',  ( -0.000000000000000000, -0.000000000000000000, -1.000000000000000000 ) ) ;
#43979=ADVANCED_FACE ( 'NONE', ( #63608 ), #17717, .T. ) ;
#43992=CARTESIAN_POINT ( 'NONE',  ( -6.880223345695647197, -142.5202692415819854, 5.500000000000000000 ) ) ;
#43996=ADVANCED_FACE ( 'NONE', ( #69600 ), #62111, .F. ) ;
#43998=AXIS2_PLACEMENT_3D ( 'NONE', #68797, #4911, #50740 ) ;
#44008=ORIENTED_EDGE ( 'NONE', *, *, #16061, .T. ) ;
#44012=CLOSED_SHELL ( 'NONE', ( #25683, #15708, #16414, #35909, #43979, #32896, #14523, #51033, #12715, #33691, #70088, #66825, #39628, #39663, #70407, #11434, #60100, #37402, #14661, #67910, #31489, #32606, #63516, #7243, #21987, #1394, #67326, #37371, #8516, #64252, #7416, #52475, #67069, #33245, #72975, #67838, #37755, #4338, #63087, #20907, #43996, #16222, #7724, #71867, #8678, #35384, #19444, #63506, #35774, #30774, #53479, #43914, #62410, #60354, #36898, #69448, #52208, #4601, #38115, #56124, #2615, #64331, #42276, #38293, #69193, #56574, #61279, #25222, #62868, #22797, #5697, #7710, #66381, #224, #38077, #16037, #31158, #12123, #72745, #24126, #46956, #72455, #52555, #24968, #7258, #4258, #14518, #14335, #48905, #10192, #35895, #49571, #53460, #53291, #20800, #35307, #68911, #13835, #21274, #16607, #62412, #74259, #16197, #61954, #64126, #64834, #25120, #39077, #72339, #74028, #5041, #47560, #66962, #33178, #41169, #58236, #43628, #56397, #74251, #65379, #68047, #36017, #70703, #25196, #44044, #71375, #46955, #22146, #24220, #62342, #1977, #49972, #60598, #16313, #10731, #20960, #61733, #20276, #57154, #36679, #70192, #2322, #50411, #37520, #62488, #20389, #36386, #8587, #20032, #11558, #11692, #27734, #22335, #7631, #43512, #54086, #7221, #21018, #20599, #64872, #9664, #46935, #53327, #67891, #42249, #52299, #30785, #13053, #67463, #71684 ) ) ;
#44014=ORIENTED_EDGE ( 'NONE', *, *, #27040, .T. ) ;
#44018=CARTESIAN_POINT ( 'NONE',  ( 22.94323693612312809, -114.6983135802921083, -5.500000000000000000 ) ) ;
#44044=ADVANCED_FACE ( 'NONE', ( #5721 ), #28997, .F. ) ;
#44047=FACE_OUTER_BOUND ( 'NONE', #20930, .T. ) ;
#44064=ORIENTED_EDGE ( 'NONE', *, *, #27040, .F. ) ;
#44074=EDGE_CURVE ( 'NONE', #36328, #18041, #53417, .T. ) ;
#44075=EDGE_LOOP ( 'NONE', ( #62132, #1602, #27384, #56226 ) ) ;
#44090=LINE ( 'NONE', #20421, #61628 ) ;
#44093=DIRECTION ( 'NONE',  ( 0.8541291221503261033, -0.5200609990133016058, 0.000000000000000000 ) ) ;
#44094=EDGE_LOOP ( 'NONE', ( #46251, #27963, #13943, #44220 ) ) ;
#44097=VERTEX_POINT ( 'NONE', #41395 ) ;
#44101=VECTOR ( 'NONE', #10631, 1000.000000000000000 ) ;
#44135=DIRECTION ( 'NONE',  ( -0.2867529058022035837, 0.9580045777625452175, 0.000000000000000000 ) ) ;
#44158=LINE ( 'NONE', #32497, #59710 ) ;
#44171=DIRECTION ( 'NONE',  ( -0.000000000000000000, -0.000000000000000000, 1.000000000000000000 ) ) ;
#44183=VERTEX_POINT ( 'NONE', #1956 ) ;
#44203=ORIENTED_EDGE ( 'NONE', *, *, #56479, .T. ) ;
#44219=DIRECTION ( 'NONE',  ( -0.000000000000000000, -0.000000000000000000, -1.000000000000000000 ) ) ;
#44220=ORIENTED_EDGE ( 'NONE', *, *, #3615, .T. ) ;
#44235=ORIENTED_EDGE ( 'NONE', *, *, #14188, .F. ) ;
#44246=EDGE_CURVE ( 'NONE', #22856, #11006, #72171, .T. ) ;
#44290=EDGE_LOOP ( 'NONE', ( #31616, #36513, #47654, #13206 ) ) ;
#44291=DIRECTION ( 'NONE',  ( -0.8225049752423776450, -0.5687579148473765889, 0.000000000000000000 ) ) ;
#44295=ORIENTED_EDGE ( 'NONE', *, *, #53316, .F. ) ;
#44309=VECTOR ( 'NONE', #55325, 1000.000000000000000 ) ;
#44318=ORIENTED_EDGE ( 'NONE', *, *, #69502, .T. ) ;
#44343=VECTOR ( 'NONE', #11741, 1000.000000000000000 ) ;
#44359=DIRECTION ( 'NONE',  ( -0.2306669878475637314, -0.9730327541852493711, 0.000000000000000000 ) ) ;
#44372=DIRECTION ( 'NONE',  ( -0.8774505977381971134, -0.4796670183876317051, 0.000000000000000000 ) ) ;
#44390=ORIENTED_EDGE ( 'NONE', *, *, #68329, .T. ) ;
#44417=VERTEX_POINT ( 'NONE', #23286 ) ;
#44423=LINE ( 'NONE', #27101, #69310 ) ;
#44467=LINE ( 'NONE', #54270, #40292 ) ;
#44474=PLANE ( 'NONE',  #19851 ) ;
#44482=EDGE_CURVE ( 'NONE', #30878, #29007, #69148, .T. ) ;
#44498=ORIENTED_EDGE ( 'NONE', *, *, #67109, .F. ) ;
#44515=DIRECTION ( 'NONE',  ( 1.000000000000000000, 0.000000000000000000, 0.000000000000000000 ) ) ;
#44533=VERTEX_POINT ( 'NONE', #22168 ) ;
#44555=EDGE_CURVE ( 'NONE', #16009, #56786, #8194, .T. ) ;
#44562=VERTEX_POINT ( 'NONE', #63885 ) ;
#44568=AXIS2_PLACEMENT_3D ( 'NONE', #2029, #24914, #36556 ) ;
#44595=ORIENTED_EDGE ( 'NONE', *, *, #59825, .F. ) ;
#44614=CARTESIAN_POINT ( 'NONE',  ( 13.36581099891334645, -139.3288669181958710, -2.500000000000000000 ) ) ;
#44618=PRODUCT_DEFINITION_SHAPE ( 'NONE', 'NONE',  #52691 ) ;
#44643=CARTESIAN_POINT ( 'NONE',  ( -30.50000000000000000, -120.0000000000000000, 5.500000000000000888 ) ) ;
#44676=VERTEX_POINT ( 'NONE', #30009 ) ;
#44686=ORIENTED_EDGE ( 'NONE', *, *, #58091, .F. ) ;
#44688=LINE ( 'NONE', #16096, #62698 ) ;
#44702=VECTOR ( 'NONE', #71128, 1000.000000000000000 ) ;
#44712=VERTEX_POINT ( 'NONE', #19474 ) ;
#44726=CARTESIAN_POINT ( 'NONE',  ( -19.90058851926621131, -132.5883508287165853, 5.500000000000000000 ) ) ;
#44727=DIRECTION ( 'NONE',  ( 0.8541291221503261033, -0.5200609990133016058, 0.000000000000000000 ) ) ;
#44759=EDGE_LOOP ( 'NONE', ( #21567, #38745, #53710, #27245 ) ) ;
#44771=EDGE_LOOP ( 'NONE', ( #7851, #58521, #51983, #36602 ) ) ;
#44802=ORIENTED_EDGE ( 'NONE', *, *, #46250, .T. ) ;
#44856=CARTESIAN_POINT ( 'NONE',  ( 8.700667342345820288, -98.11853780484867116, 5.500000000000000000 ) ) ;
#44877=ORIENTED_EDGE ( 'NONE', *, *, #25811, .T. ) ;
#44897=DIRECTION ( 'NONE',  ( -0.1850432970638667129, 0.9827303690289281857, 0.000000000000000000 ) ) ;
#44923=FACE_OUTER_BOUND ( 'NONE', #65493, .T. ) ;
#44973=EDGE_CURVE ( 'NONE', #31529, #105, #4816, .T. ) ;
#44980=LINE ( 'NONE', #44614, #7346 ) ;
#44981=DIRECTION ( 'NONE',  ( -0.9918136447140104561, 0.1276937514489679681, 0.000000000000000000 ) ) ;
#44988=CARTESIAN_POINT ( 'NONE',  ( -103.9230484541323705, -180.0000000000004832, -5.500000000000000000 ) ) ;
#45040=PLANE ( 'NONE',  #46594 ) ;
#45091=LINE ( 'NONE', #15763, #14775 ) ;
#45094=DIRECTION ( 'NONE',  ( 0.9827303690289279636, 0.1850432970638682395, 0.000000000000000000 ) ) ;
#45100=CARTESIAN_POINT ( 'NONE',  ( 30.50000000000000000, -120.0000000000000000, -2.500000000000000000 ) ) ;
#45117=AXIS2_PLACEMENT_3D ( 'NONE', #49865, #32941, #16038 ) ;
#45119=CARTESIAN_POINT ( 'NONE',  ( 2.047646702416564768, -96.54137380445985173, 5.500000000000000000 ) ) ;
#45122=AXIS2_PLACEMENT_3D ( 'NONE', #14458, #15193, #19720 ) ;
#45134=VERTEX_POINT ( 'NONE', #58141 ) ;
#45140=ORIENTED_EDGE ( 'NONE', *, *, #7869, .F. ) ;
#45166=DIRECTION ( 'NONE',  ( -0.000000000000000000, -0.000000000000000000, -1.000000000000000000 ) ) ;
#45180=FACE_OUTER_BOUND ( 'NONE', #27545, .T. ) ;
#45189=DIRECTION ( 'NONE',  ( -0.8225049752423776450, -0.5687579148473765889, 0.000000000000000000 ) ) ;
#45193=CARTESIAN_POINT ( 'NONE',  ( 1.474095553543393056, -119.7224350544041869, 2.500000000000000000 ) ) ;
#45198=DIRECTION ( 'NONE',  ( 0.000000000000000000, 0.000000000000000000, 1.000000000000000000 ) ) ;
#45213=ORIENTED_EDGE ( 'NONE', *, *, #29332, .F. ) ;
#45218=CARTESIAN_POINT ( 'NONE',  ( -24.94940289813038703, -237.3777120880567963, -5.500000000000000000 ) ) ;
#45219=VERTEX_POINT ( 'NONE', #43730 ) ;
#45237=VERTEX_POINT ( 'NONE', #50075 ) ;
#45267=EDGE_CURVE ( 'NONE', #63916, #38750, #38071, .T. ) ;
#45303=VECTOR ( 'NONE', #60749, 1000.000000000000114 ) ;
#45310=LINE ( 'NONE', #16350, #29149 ) ;
#45322=PLANE ( 'NONE',  #42984 ) ;
#45324=VECTOR ( 'NONE', #67245, 1000.000000000000114 ) ;
#45332=EDGE_CURVE ( 'NONE', #44183, #40306, #5366, .T. ) ;
#45350=DIRECTION ( 'NONE',  ( 0.7950889364178796992, -0.6064928550163511956, 0.000000000000000000 ) ) ;
#45420=DIRECTION ( 'NONE',  ( -0.1850432970638682395, 0.9827303690289280746, 0.000000000000000000 ) ) ;
#45470=DIRECTION ( 'NONE',  ( -0.7273375899149793211, 0.6862798483830554463, 0.000000000000000000 ) ) ;
#45480=CARTESIAN_POINT ( 'NONE',  ( 20.85212586905262100, -130.9402397935870965, 5.500000000000000000 ) ) ;
#45489=DIRECTION ( 'NONE',  ( 0.9997280174009349762, -0.02332147558787671729, 0.000000000000000000 ) ) ;
#45507=PLANE ( 'NONE',  #63541 ) ;
#45549=LINE ( 'NONE', #10949, #930 ) ;
#45578=CARTESIAN_POINT ( 'NONE',  ( 0.000000000000000000, -120.0000000000000000, 2.500000000000000000 ) ) ;
#45581=CARTESIAN_POINT ( 'NONE',  ( -26.29030328629083968, -123.6496510949466341, 5.500000000000000000 ) ) ;
#45584=EDGE_CURVE ( 'NONE', #26049, #17019, #18461, .T. ) ;
#45592=VERTEX_POINT ( 'NONE', #35747 ) ;
#45593=VECTOR ( 'NONE', #14195, 999.9999999999998863 ) ;
#45628=DIRECTION ( 'NONE',  ( 0.9435911131814398445, -0.3311129884571295534, 0.000000000000000000 ) ) ;
#45647=CARTESIAN_POINT ( 'NONE',  ( -7.572224309238338336, -145.4393675041377492, 5.500000000000000000 ) ) ;
#45660=PLANE ( 'NONE',  #21103 ) ;
#45706=CARTESIAN_POINT ( 'NONE',  ( -14.87942725330654348, -141.9795960975983178, 5.500000000000000000 ) ) ;
#45726=VERTEX_POINT ( 'NONE', #71805 ) ;
#45742=LINE ( 'NONE', #74285, #72041 ) ;
#45752=DIRECTION ( 'NONE',  ( 0.4279312458753000703, 0.9038112904824842087, 0.000000000000000000 ) ) ;
#45769=EDGE_CURVE ( 'NONE', #19317, #21360, #35935, .T. ) ;
#45777=VECTOR ( 'NONE', #19347, 1000.000000000000000 ) ;
#45779=CARTESIAN_POINT ( 'NONE',  ( 18.80329974962065265, -105.8248132807389084, -5.500000000000000000 ) ) ;
#45780=ORIENTED_EDGE ( 'NONE', *, *, #59590, .F. ) ;
#45787=DIRECTION ( 'NONE',  ( -0.9730327541852497042, 0.2306669878475623159, 0.000000000000000000 ) ) ;
#45798=EDGE_CURVE ( 'NONE', #70524, #26348, #43152, .T. ) ;
#45816=AXIS2_PLACEMENT_3D ( 'NONE', #70009, #51984, #904 ) ;
#45824=ORIENTED_EDGE ( 'NONE', *, *, #54155, .T. ) ;
#45828=DIRECTION ( 'NONE',  ( 0.2306669878475623159, 0.9730327541852497042, -0.000000000000000000 ) ) ;
#45863=LINE ( 'NONE', #68787, #67008 ) ;
#45871=ORIENTED_EDGE ( 'NONE', *, *, #47435, .F. ) ;
#45884=VECTOR ( 'NONE', #48210, 1000.000000000000000 ) ;
#45901=VERTEX_POINT ( 'NONE', #48004 ) ;
#45922=LINE ( 'NONE', #4964, #43572 ) ;
#45942=ORIENTED_EDGE ( 'NONE', *, *, #63766, .T. ) ;
#45950=EDGE_CURVE ( 'NONE', #61799, #7483, #13409, .T. ) ;
#45951=DIRECTION ( 'NONE',  ( 0.3853207896976533209, -0.9227826878668545785, 0.000000000000000000 ) ) ;
#45961=ORIENTED_EDGE ( 'NONE', *, *, #68058, .F. ) ;
#45964=FACE_OUTER_BOUND ( 'NONE', #16628, .T. ) ;
#45974=EDGE_LOOP ( 'NONE', ( #54010, #72574, #41147, #54859 ) ) ;
#45975=EDGE_LOOP ( 'NONE', ( #27093, #63907, #47268, #54765 ) ) ;
#45996=DIRECTION ( 'NONE',  ( 0.9918136447140101231, -0.1276937514489694114, 0.000000000000000000 ) ) ;
#46000=EDGE_CURVE ( 'NONE', #27087, #70823, #50959, .T. ) ;
#46031=DIRECTION ( 'NONE',  ( -0.8225049752423791993, -0.5687579148473745905, 0.000000000000000000 ) ) ;
#46043=DIRECTION ( 'NONE',  ( 0.9038112904824853189, -0.4279312458752977388, 0.000000000000000000 ) ) ;
#46069=ORIENTED_EDGE ( 'NONE', *, *, #34357, .F. ) ;
#46080=LINE ( 'NONE', #23889, #16924 ) ;
#46095=DIRECTION ( 'NONE',  ( -0.3853207896976533764, 0.9227826878668546895, 0.000000000000000000 ) ) ;
#46106=DIRECTION ( 'NONE',  ( 1.000000000000000000, 0.000000000000000000, 0.000000000000000000 ) ) ;
#46109=DIRECTION ( 'NONE',  ( 0.5200609990132993854, 0.8541291221503275466, 0.000000000000000000 ) ) ;
#46117=ORIENTED_EDGE ( 'NONE', *, *, #19028, .T. ) ;
#46137=ORIENTED_EDGE ( 'NONE', *, *, #62141, .T. ) ;
#46148=ORIENTED_EDGE ( 'NONE', *, *, #15773, .F. ) ;
#46172=VERTEX_POINT ( 'NONE', #982 ) ;
#46183=CARTESIAN_POINT ( 'NONE',  ( -7.572224309238338336, -145.4393675041377492, 5.500000000000000000 ) ) ;
#46188=VECTOR ( 'NONE', #66998, 1000.000000000000000 ) ;
#46194=CARTESIAN_POINT ( 'NONE',  ( -10.43921258969510824, -98.89258801967538659, 5.500000000000000000 ) ) ;
#46223=ORIENTED_EDGE ( 'NONE', *, *, #3402, .F. ) ;
#46240=ORIENTED_EDGE ( 'NONE', *, *, #36054, .F. ) ;
#46244=CARTESIAN_POINT ( 'NONE',  ( -10.43921258969510824, -98.89258801967538659, 5.500000000000000000 ) ) ;
#46250=EDGE_CURVE ( 'NONE', #35224, #14992, #17488, .T. ) ;
#46251=ORIENTED_EDGE ( 'NONE', *, *, #62688, .F. ) ;
#46305=FACE_OUTER_BOUND ( 'NONE', #39576, .T. ) ;
#46309=VERTEX_POINT ( 'NONE', #13324 ) ;
#46316=EDGE_CURVE ( 'NONE', #13677, #28951, #48653, .T. ) ;
#46378=ORIENTED_EDGE ( 'NONE', *, *, #57877, .F. ) ;
#46384=PLANE ( 'NONE',  #38126 ) ;
#46387=FILL_AREA_STYLE ('',( #2040 ) ) ;
#46409=VECTOR ( 'NONE', #28543, 1000.000000000000000 ) ;
#46443=EDGE_CURVE ( 'NONE', #51420, #12142, #15548, .T. ) ;
#46458=DIRECTION ( 'NONE',  ( 0.9997280174009348652, -0.02332147558787931590, 0.000000000000000000 ) ) ;
#46466=CARTESIAN_POINT ( 'NONE',  ( 0.000000000000000000, -120.0000000000000000, 2.500000000000000000 ) ) ;
#46475=VECTOR ( 'NONE', #52050, 1000.000000000000114 ) ;
#46531=DIRECTION ( 'NONE',  ( -0.6064928550163524168, -0.7950889364178789220, 0.000000000000000000 ) ) ;
#46548=VERTEX_POINT ( 'NONE', #15170 ) ;
#46575=CARTESIAN_POINT ( 'NONE',  ( 13.36581099891334645, -139.3288669181958710, 2.500000000000000000 ) ) ;
#46576=ORIENTED_EDGE ( 'NONE', *, *, #45584, .T. ) ;
#46594=AXIS2_PLACEMENT_3D ( 'NONE', #4455, #27738, #44291 ) ;
#46598=VECTOR ( 'NONE', #7817, 1000.000000000000000 ) ;
#46607=DIRECTION ( 'NONE',  ( 0.9580045777625458836, 0.2867529058022011412, 0.000000000000000000 ) ) ;
#46635=CARTESIAN_POINT ( 'NONE',  ( -22.17439115976385366, -112.2188447712574799, -2.500000000000000000 ) ) ;
#46646=DIRECTION ( 'NONE',  ( -0.6064928550163533050, -0.7950889364178781449, 0.000000000000000000 ) ) ;
#46657=CARTESIAN_POINT ( 'NONE',  ( -24.50849501662245800, -109.8101191361138831, 5.500000000000000000 ) ) ;
#46676=ORIENTED_EDGE ( 'NONE', *, *, #18535, .F. ) ;
#46700=EDGE_CURVE ( 'NONE', #13957, #15423, #22682, .T. ) ;
#46702=CARTESIAN_POINT ( 'NONE',  ( -1.384174031800281979, -120.5779811845464735, 2.500000000000000000 ) ) ;
#46703=ORIENTED_EDGE ( 'NONE', *, *, #18464, .F. ) ;
#46707=ORIENTED_EDGE ( 'NONE', *, *, #9173, .F. ) ;
#46729=DIRECTION ( 'NONE',  ( -0.4279312458753000703, -0.9038112904824842087, 0.000000000000000000 ) ) ;
#46736=LINE ( 'NONE', #70014, #39815 ) ;
#46744=VECTOR ( 'NONE', #36484, 1000.000000000000114 ) ;
#46755=CARTESIAN_POINT ( 'NONE',  ( 0.000000000000000000, -120.0000000000000000, -5.500000000000000000 ) ) ;
#46762=EDGE_CURVE ( 'NONE', #26154, #20073, #3099, .T. ) ;
#46773=LINE ( 'NONE', #64431, #10659 ) ;
#46790=EDGE_LOOP ( 'NONE', ( #67394, #35856, #28209, #27238 ) ) ;
#46803=VERTEX_POINT ( 'NONE', #37296 ) ;
#46818=ORIENTED_EDGE ( 'NONE', *, *, #62993, .T. ) ;
#46841=ORIENTED_EDGE ( 'NONE', *, *, #7067, .T. ) ;
#46872=VECTOR ( 'NONE', #60807, 1000.000000000000000 ) ;
#46875=CARTESIAN_POINT ( 'NONE',  ( -7.670864526094549163, -97.73662565058241114, 5.500000000000000000 ) ) ;
#46883=CARTESIAN_POINT ( 'NONE',  ( 2.874421927457452952, -143.3717286177755739, 5.500000000000000000 ) ) ;
#46889=EDGE_LOOP ( 'NONE', ( #51027, #23317, #10252, #6519 ) ) ;
#46917=VERTEX_POINT ( 'NONE', #66236 ) ;
#46935=ADVANCED_FACE ( 'NONE', ( #73327, #4945 ), #9073, .F. ) ;
#46955=ADVANCED_FACE ( 'NONE', ( #15077 ), #21447, .F. ) ;
#46956=ADVANCED_FACE ( 'NONE', ( #21080 ), #26722, .F. ) ;
#46968=ORIENTED_EDGE ( 'NONE', *, *, #14610, .F. ) ;
#46976=ORIENTED_EDGE ( 'NONE', *, *, #10696, .T. ) ;
#46993=VERTEX_POINT ( 'NONE', #27090 ) ;
#47037=CARTESIAN_POINT ( 'NONE',  ( 13.83832728059186046, -142.6495187161941089, 5.500000000000000000 ) ) ;
#47056=DIRECTION ( 'NONE',  ( 0.000000000000000000, 0.000000000000000000, 1.000000000000000000 ) ) ;
#47067=ORIENTED_EDGE ( 'NONE', *, *, #17720, .F. ) ;
#47091=DIRECTION ( 'NONE',  ( 0.9966891607226785466, 0.08130631524009969413, 0.000000000000000000 ) ) ;
#47103=CARTESIAN_POINT ( 'NONE',  ( 18.80329974962065265, -105.8248132807389084, 5.500000000000000000 ) ) ;
#47111=DIRECTION ( 'NONE',  ( -0.8774505977381983346, -0.4796670183876294291, 0.000000000000000000 ) ) ;
#47119=LINE ( 'NONE', #31650, #44702 ) ;
#47131=DIRECTION ( 'NONE',  ( 0.5687579148473744795, -0.8225049752423790883, 0.000000000000000000 ) ) ;
#47139=EDGE_LOOP ( 'NONE', ( #72725, #48919, #61769, #70978 ) ) ;
#47167=VERTEX_POINT ( 'NONE', #30792 ) ;
#47169=LINE ( 'NONE', #70078, #8274 ) ;
#47208=VECTOR ( 'NONE', #48853, 1000.000000000000114 ) ;
#47216=PLANE ( 'NONE',  #14837 ) ;
#47224=ORIENTED_EDGE ( 'NONE', *, *, #56126, .T. ) ;
#47268=ORIENTED_EDGE ( 'NONE', *, *, #60554, .F. ) ;
#47290=CARTESIAN_POINT ( 'NONE',  ( 16.30584220631899228, -140.9432449716519784, 2.500000000000000000 ) ) ;
#47312=AXIS2_PLACEMENT_3D ( 'NONE', #27445, #37273, #32708 ) ;
#47322=DIRECTION ( 'NONE',  ( -0.1045284632676436315, -0.9945218953682742891, 0.000000000000000000 ) ) ;
#47368=EDGE_LOOP ( 'NONE', ( #23129, #35297, #13222, #16473 ) ) ;
#47370=CARTESIAN_POINT ( 'NONE',  ( 2.117611129180199558, -93.54218975225703048, -5.500000000000000000 ) ) ;
#47380=CARTESIAN_POINT ( 'NONE',  ( 12.13205353604972991, -140.1820037904669789, 5.500000000000000000 ) ) ;
#47381=EDGE_CURVE ( 'NONE', #37554, #32596, #44980, .T. ) ;
#47382=CARTESIAN_POINT ( 'NONE',  ( -70.53423027509626309, -217.0820393249940423, -5.500000000000000000 ) ) ;
#47393=EDGE_CURVE ( 'NONE', #54089, #37730, #16777, .T. ) ;
#47419=EDGE_CURVE ( 'NONE', #11723, #51387, #33298, .T. ) ;
#47435=EDGE_CURVE ( 'NONE', #20698, #47697, #14626, .T. ) ;
#47474=VECTOR ( 'NONE', #73564, 1000.000000000000000 ) ;
#47478=DIRECTION ( 'NONE',  ( -0.000000000000000000, -0.000000000000000000, -1.000000000000000000 ) ) ;
#47488=DIRECTION ( 'NONE',  ( 0.4796670183876304283, -0.8774505977381978905, 0.000000000000000000 ) ) ;
#47493=CARTESIAN_POINT ( 'NONE',  ( -22.53294031248082163, -134.0273518838794757, 5.500000000000000000 ) ) ;
#47497=( LENGTH_UNIT ( ) NAMED_UNIT ( * ) SI_UNIT ( .MILLI., .METRE. ) );
#47513=VECTOR ( 'NONE', #43779, 1000.000000000000000 ) ;
#47515=EDGE_CURVE ( 'NONE', #16806, #57541, #52086, .T. ) ;
#47520=AXIS2_PLACEMENT_3D ( 'NONE', #62287, #43883, #27302 ) ;
#47534=ORIENTED_EDGE ( 'NONE', *, *, #62909, .T. ) ;
#47559=DIRECTION ( 'NONE',  ( -0.000000000000000000, -0.000000000000000000, -1.000000000000000000 ) ) ;
#47560=ADVANCED_FACE ( 'NONE', ( #24624 ), #70466, .F. ) ;
#47564=EDGE_LOOP ( 'NONE', ( #12551, #11389, #23315, #48793 ) ) ;
#47567=LINE ( 'NONE', #18979, #6375 ) ;
#47568=LINE ( 'NONE', #1748, #6554 ) ;
#47582=LINE ( 'NONE', #70487, #43072 ) ;
#47602=CARTESIAN_POINT ( 'NONE',  ( 2.874421927457452952, -143.3717286177755739, 2.500000000000000000 ) ) ;
#47613=VECTOR ( 'NONE', #53443, 1000.000000000000114 ) ;
#47616=ORIENTED_EDGE ( 'NONE', *, *, #20653, .F. ) ;
#47621=VECTOR ( 'NONE', #6871, 1000.000000000000000 ) ;
#47626=EDGE_CURVE ( 'NONE', #14636, #33066, #8454, .T. ) ;
#47654=ORIENTED_EDGE ( 'NONE', *, *, #71813, .F. ) ;
#47697=VERTEX_POINT ( 'NONE', #59585 ) ;
#47706=DIRECTION ( 'NONE',  ( 1.000000000000000000, 0.000000000000000000, 0.000000000000000000 ) ) ;
#47723=LINE ( 'NONE', #60415, #36610 ) ;
#47728=VECTOR ( 'NONE', #13635, 1000.000000000000000 ) ;
#47730=DIRECTION ( 'NONE',  ( -0.8541291221503275466, 0.5200609990132993854, 0.000000000000000000 ) ) ;
#47738=ORIENTED_EDGE ( 'NONE', *, *, #49410, .T. ) ;
#47741=CARTESIAN_POINT ( 'NONE',  ( 6.377742925735834234, -145.7647898336707897, -2.500000000000000000 ) ) ;
#47744=AXIS2_PLACEMENT_3D ( 'NONE', #66117, #2978, #2624 ) ;
#47756=DIRECTION ( 'NONE',  ( 0.6064928550163524168, 0.7950889364178788110, 0.000000000000000000 ) ) ;
#47764=DIRECTION ( 'NONE',  ( 0.000000000000000000, 0.000000000000000000, 1.000000000000000000 ) ) ;
#47768=CARTESIAN_POINT ( 'NONE',  ( -21.33958957442910886, -129.9559990355020034, 2.500000000000000000 ) ) ;
#47794=LINE ( 'NONE', #25599, #58034 ) ;
#47804=VECTOR ( 'NONE', #42977, 1000.000000000000114 ) ;
#47837=DIRECTION ( 'NONE',  ( 0.02332147558787931590, 0.9997280174009348652, 0.000000000000000000 ) ) ;
#47842=CARTESIAN_POINT ( 'NONE',  ( 22.51310757741980240, -113.2613067136482101, 2.500000000000000000 ) ) ;
#47844=PLANE ( 'NONE',  #42212 ) ;
#47854=SURFACE_SIDE_STYLE ('',( #57679 ) ) ;
#47881=VECTOR ( 'NONE', #50721, 1000.000000000000000 ) ;
#47886=ORIENTED_EDGE ( 'NONE', *, *, #17510, .F. ) ;
#47898=VECTOR ( 'NONE', #52265, 1000.000000000000114 ) ;
#47935=DIRECTION ( 'NONE',  ( -0.9038112904824853189, 0.4279312458752976833, 0.000000000000000000 ) ) ;
#47986=CARTESIAN_POINT ( 'NONE',  ( 24.95699195200416654, -110.9640411295978595, 5.500000000000000000 ) ) ;
#48004=CARTESIAN_POINT ( 'NONE',  ( -21.67772167707813935, -110.8034581014852762, -5.500000000000000000 ) ) ;
#48012=LINE ( 'NONE', #31075, #7382 ) ;
#48054=EDGE_CURVE ( 'NONE', #11355, #11947, #46736, .T. ) ;
#48057=ORIENTED_EDGE ( 'NONE', *, *, #62688, .T. ) ;
#48058=CARTESIAN_POINT ( 'NONE',  ( 119.3426274441929280, -132.5434155921172419, 5.500000000000000000 ) ) ;
#48069=VECTOR ( 'NONE', #45951, 1000.000000000000114 ) ;
#48073=LINE ( 'NONE', #42436, #72390 ) ;
#48120=VECTOR ( 'NONE', #50334, 1000.000000000000000 ) ;
#48136=EDGE_CURVE ( 'NONE', #69025, #62465, #65510, .T. ) ;
#48137=UNCERTAINTY_MEASURE_WITH_UNIT (LENGTH_MEASURE( 1.000000000000000082E-05 ), #12455, 'distance_accuracy_value', 'NONE');
#48152=FACE_OUTER_BOUND ( 'NONE', #62271, .T. ) ;
#48154=AXIS2_PLACEMENT_3D ( 'NONE', #32467, #73051, #44515 ) ;
#48167=VERTEX_POINT ( 'NONE', #48932 ) ;
#48172=DIRECTION ( 'NONE',  ( -0.000000000000000000, -0.000000000000000000, -1.000000000000000000 ) ) ;
#48173=ORIENTED_EDGE ( 'NONE', *, *, #16722, .F. ) ;
#48185=DIRECTION ( 'NONE',  ( 0.6862798483830554463, 0.7273375899149793211, -0.000000000000000000 ) ) ;
#48196=EDGE_CURVE ( 'NONE', #32752, #12079, #36182, .T. ) ;
#48202=DIRECTION ( 'NONE',  ( 0.7585478161175716050, 0.6516173805718067369, 0.000000000000000000 ) ) ;
#48210=DIRECTION ( 'NONE',  ( -0.000000000000000000, -0.000000000000000000, -1.000000000000000000 ) ) ;
#48258=ORIENTED_EDGE ( 'NONE', *, *, #54821, .T. ) ;
#48293=DIRECTION ( 'NONE',  ( -0.5687579148473752566, 0.8225049752423786442, 0.000000000000000000 ) ) ;
#48320=CARTESIAN_POINT ( 'NONE',  ( 0.000000000000000000, 0.000000000000000000, 0.000000000000000000 ) ) ;
#48323=EDGE_CURVE ( 'NONE', #47697, #49297, #49307, .T. ) ;
#48329=ORIENTED_EDGE ( 'NONE', *, *, #60635, .F. ) ;
#48337=LINE ( 'NONE', #395, #59839 ) ;
#48369=CARTESIAN_POINT ( 'NONE',  ( 23.49916127795269460, -121.5130826919798039, 5.500000000000000000 ) ) ;
#48420=VECTOR ( 'NONE', #60387, 1000.000000000000000 ) ;
#48431=FACE_OUTER_BOUND ( 'NONE', #41889, .T. ) ;
#48463=CARTESIAN_POINT ( 'NONE',  ( 11.41210121379328335, -99.40233154247455616, 5.500000000000000000 ) ) ;
#48501=DIRECTION ( 'NONE',  ( -0.9580045777625459946, -0.2867529058022011412, 0.000000000000000000 ) ) ;
#48504=DIRECTION ( 'NONE',  ( -0.9227826878668540234, -0.3853207896976547642, 0.000000000000000000 ) ) ;
#48540=LINE ( 'NONE', #53808, #47613 ) ;
#48548=ORIENTED_EDGE ( 'NONE', *, *, #4513, .F. ) ;
#48551=ORIENTED_EDGE ( 'NONE', *, *, #54236, .T. ) ;
#48607=VECTOR ( 'NONE', #7425, 1000.000000000000000 ) ;
#48616=ORIENTED_EDGE ( 'NONE', *, *, #27471, .F. ) ;
#48648=CARTESIAN_POINT ( 'NONE',  ( -17.26469406256017791, -140.1601175325492648, 5.500000000000000000 ) ) ;
#48652=AXIS2_PLACEMENT_3D ( 'NONE', #65332, #31096, #8554 ) ;
#48653=LINE ( 'NONE', #31350, #61173 ) ;
#48661=VERTEX_POINT ( 'NONE', #18294 ) ;
#48684=PLANE ( 'NONE',  #30860 ) ;
#48704=ORIENTED_EDGE ( 'NONE', *, *, #30678, .F. ) ;
#48705=VECTOR ( 'NONE', #47111, 1000.000000000000114 ) ;
#48717=FACE_OUTER_BOUND ( 'NONE', #53369, .T. ) ;
#48732=VERTEX_POINT ( 'NONE', #40492 ) ;
#48742=VECTOR ( 'NONE', #52735, 1000.000000000000114 ) ;
#48743=CARTESIAN_POINT ( 'NONE',  ( 0.1219594728601484379, -121.4950337410840149, 2.500000000000000000 ) ) ;
#48757=VECTOR ( 'NONE', #62482, 1000.000000000000000 ) ;
#48793=ORIENTED_EDGE ( 'NONE', *, *, #33635, .T. ) ;
#48806=LINE ( 'NONE', #13112, #62373 ) ;
#48825=ORIENTED_EDGE ( 'NONE', *, *, #28423, .T. ) ;
#48827=DIRECTION ( 'NONE',  ( -0.9918136447140101231, 0.1276937514489694114, 0.000000000000000000 ) ) ;
#48832=EDGE_LOOP ( 'NONE', ( #71756, #10298, #52484, #8609 ) ) ;
#48838=DIRECTION ( 'NONE',  ( -0.000000000000000000, -0.000000000000000000, 1.000000000000000000 ) ) ;
#48840=ORIENTED_EDGE ( 'NONE', *, *, #37207, .T. ) ;
#48844=FACE_OUTER_BOUND ( 'NONE', #29389, .T. ) ;
#48845=AXIS2_PLACEMENT_3D ( 'NONE', #47382, #54495, #54135 ) ;
#48847=DIRECTION ( 'NONE',  ( -0.9435911131814395114, 0.3311129884571304971, 0.000000000000000000 ) ) ;
#48853=DIRECTION ( 'NONE',  ( 0.6516173805718079581, -0.7585478161175704948, 0.000000000000000000 ) ) ;
#48860=AXIS2_PLACEMENT_3D ( 'NONE', #65448, #47764, #71057 ) ;
#48875=LINE ( 'NONE', #50356, #12167 ) ;
#48905=ADVANCED_FACE ( 'NONE', ( #48717 ), #3256, .F. ) ;
#48919=ORIENTED_EDGE ( 'NONE', *, *, #33415, .F. ) ;
#48932=CARTESIAN_POINT ( 'NONE',  ( 26.09152095774781799, -124.8716048804687375, -2.500000000000000444 ) ) ;
#48951=LINE ( 'NONE', #66272, #14115 ) ;
#48981=LINE ( 'NONE', #66660, #40621 ) ;
#49036=EDGE_CURVE ( 'NONE', #14738, #33943, #43051, .T. ) ;
#49062=VERTEX_POINT ( 'NONE', #59979 ) ;
#49071=EDGE_CURVE ( 'NONE', #4157, #7707, #47567, .T. ) ;
#49090=ORIENTED_EDGE ( 'NONE', *, *, #7575, .F. ) ;
#49115=DIRECTION ( 'NONE',  ( 0.7273375899149802093, -0.6862798483830544471, 0.000000000000000000 ) ) ;
#49118=VERTEX_POINT ( 'NONE', #36280 ) ;
#49134=EDGE_CURVE ( 'NONE', #31970, #57738, #19724, .T. ) ;
#49166=LINE ( 'NONE', #72091, #7912 ) ;
#49179=ORIENTED_EDGE ( 'NONE', *, *, #50823, .F. ) ;
#49221=DIRECTION ( 'NONE',  ( 0.000000000000000000, 0.000000000000000000, 1.000000000000000000 ) ) ;
#49226=LINE ( 'NONE', #27400, #18157 ) ;
#49257=DIRECTION ( 'NONE',  ( 0.5687579148473743684, -0.8225049752423791993, 0.000000000000000000 ) ) ;
#49272=VECTOR ( 'NONE', #25816, 1000.000000000000000 ) ;
#49297=VERTEX_POINT ( 'NONE', #49415 ) ;
#49304=DIRECTION ( 'NONE',  ( -0.000000000000000000, -0.000000000000000000, -1.000000000000000000 ) ) ;
#49307=LINE ( 'NONE', #60963, #18219 ) ;
#49309=LINE ( 'NONE', #60250, #62361 ) ;
#49333=CARTESIAN_POINT ( 'NONE',  ( 2.874421927457452952, -143.3717286177755739, -2.500000000000000000 ) ) ;
#49337=DIRECTION ( 'NONE',  ( -0.08130631524009862554, 0.9966891607226787686, 0.000000000000000000 ) ) ;
#49351=DIRECTION ( 'NONE',  ( 0.8774505977381978905, 0.4796670183876304283, 0.000000000000000000 ) ) ;
#49353=DIRECTION ( 'NONE',  ( -0.1276937514489679404, -0.9918136447140103451, 0.000000000000000000 ) ) ;
#49362=ORIENTED_EDGE ( 'NONE', *, *, #15505, .F. ) ;
#49372=COLOUR_RGB ( '', 0.09019608, 0.27058824, 0.51372549) ;
#49410=EDGE_CURVE ( 'NONE', #23556, #2800, #40360, .T. ) ;
#49413=DIRECTION ( 'NONE',  ( -0.000000000000000000, -0.000000000000000000, -1.000000000000000000 ) ) ;
#49415=CARTESIAN_POINT ( 'NONE',  ( 12.69589495141918611, -96.69089767102708777, -5.500000000000000000 ) ) ;
#49418=ORIENTED_EDGE ( 'NONE', *, *, #11159, .F. ) ;
#49424=LINE ( 'NONE', #71228, #6987 ) ;
#49456=CARTESIAN_POINT ( 'NONE',  ( -0.9515373497862389396, -96.47140937769621871, 5.500000000000000000 ) ) ;
#49489=VERTEX_POINT ( 'NONE', #25555 ) ;
#49505=EDGE_CURVE ( 'NONE', #57738, #2902, #3036, .T. ) ;
#49537=CARTESIAN_POINT ( 'NONE',  ( 22.94323693612312809, -114.6983135802921083, 2.500000000000000000 ) ) ;
#49547=ORIENTED_EDGE ( 'NONE', *, *, #31759, .F. ) ;
#49557=ORIENTED_EDGE ( 'NONE', *, *, #2361, .F. ) ;
#49566=LINE ( 'NONE', #72494, #38443 ) ;
#49571=ADVANCED_FACE ( 'NONE', ( #59782 ), #14644, .F. ) ;
#49612=ORIENTED_EDGE ( 'NONE', *, *, #39381, .F. ) ;
#49627=ORIENTED_EDGE ( 'NONE', *, *, #63676, .T. ) ;
#49631=CARTESIAN_POINT ( 'NONE',  ( 16.84844760790522855, -103.5491698323862124, 5.500000000000000000 ) ) ;
#49659=EDGE_CURVE ( 'NONE', #11006, #55103, #45091, .T. ) ;
#49664=DIRECTION ( 'NONE',  ( -0.9580045777625452175, -0.2867529058022035837, 0.000000000000000000 ) ) ;
#49671=DIRECTION ( 'NONE',  ( -0.000000000000000000, -0.000000000000000000, -1.000000000000000000 ) ) ;
#49690=EDGE_CURVE ( 'NONE', #53859, #64729, #10872, .T. ) ;
#49692=EDGE_LOOP ( 'NONE', ( #38540, #63256, #14619, #53802 ) ) ;
#49719=ORIENTED_EDGE ( 'NONE', *, *, #54555, .T. ) ;
#49722=DIRECTION ( 'NONE',  ( -0.000000000000000000, -0.000000000000000000, -1.000000000000000000 ) ) ;
#49733=ORIENTED_EDGE ( 'NONE', *, *, #35168, .T. ) ;
#49740=LINE ( 'NONE', #15915, #52336 ) ;
#49755=AXIS2_PLACEMENT_3D ( 'NONE', #41399, #40665, #7191 ) ;
#49772=DIRECTION ( 'NONE',  ( -0.7273375899149802093, 0.6862798483830544471, 0.000000000000000000 ) ) ;
#49791=DIRECTION ( 'NONE',  ( 1.000000000000000000, 0.000000000000000000, 0.000000000000000000 ) ) ;
#49827=DIRECTION ( 'NONE',  ( 0.6064928550163524168, 0.7950889364178788110, 0.000000000000000000 ) ) ;
#49837=ORIENTED_EDGE ( 'NONE', *, *, #54427, .T. ) ;
#49840=CARTESIAN_POINT ( 'NONE',  ( -26.53422223201112828, -120.6595836127786043, 5.500000000000000000 ) ) ;
#49841=EDGE_CURVE ( 'NONE', #48661, #63983, #29613, .T. ) ;
#49843=AXIS2_PLACEMENT_3D ( 'NONE', #43907, #37521, #31490 ) ;
#49850=CARTESIAN_POINT ( 'NONE',  ( 6.377742925735834234, -145.7647898336708181, 5.500000000000000000 ) ) ;
#49865=CARTESIAN_POINT ( 'NONE',  ( 0.000000000000000000, -120.0000000000000000, 2.500000000000000000 ) ) ;
#49876=LINE ( 'NONE', #40462, #39417 ) ;
#49889=DIRECTION ( 'NONE',  ( -0.6516173805718079581, 0.7585478161175706058, 0.000000000000000000 ) ) ;
#49896=CARTESIAN_POINT ( 'NONE',  ( -7.572224309238338336, -145.4393675041377492, -5.500000000000000000 ) ) ;
#49913=ORIENTED_EDGE ( 'NONE', *, *, #54257, .T. ) ;
#49930=VECTOR ( 'NONE', #36923, 1000.000000000000227 ) ;
#49972=ADVANCED_FACE ( 'NONE', ( #20191 ), #43889, .F. ) ;
#49982=CARTESIAN_POINT ( 'NONE',  ( 13.83832728059186046, -142.6495187161941089, 2.500000000000000000 ) ) ;
#50007=ORIENTED_EDGE ( 'NONE', *, *, #60274, .T. ) ;
#50012=ORIENTED_EDGE ( 'NONE', *, *, #42374, .T. ) ;
#50023=EDGE_CURVE ( 'NONE', #48167, #26154, #19456, .T. ) ;
#50051=DIRECTION ( 'NONE',  ( 0.9827303690289279636, 0.1850432970638682395, -0.000000000000000000 ) ) ;
#50075=CARTESIAN_POINT ( 'NONE',  ( 21.85433023846371370, -135.0628101570779620, -2.500000000000000444 ) ) ;
#50088=VERTEX_POINT ( 'NONE', #67926 ) ;
#50125=LINE ( 'NONE', #45647, #64704 ) ;
#50135=DIRECTION ( 'NONE',  ( -1.000000000000000000, 0.000000000000000000, 0.000000000000000000 ) ) ;
#50143=CARTESIAN_POINT ( 'NONE',  ( -8.826826895187510402, -94.96827758698185562, 2.500000000000000000 ) ) ;
#50176=VECTOR ( 'NONE', #49413, 1000.000000000000000 ) ;
#50186=LINE ( 'NONE', #23764, #39380 ) ;
#50189=ORIENTED_EDGE ( 'NONE', *, *, #37534, .F. ) ;
#50202=EDGE_LOOP ( 'NONE', ( #60253, #18850, #42415, #48825 ) ) ;
#50209=AXIS2_PLACEMENT_3D ( 'NONE', #62795, #21402, #5642 ) ;
#50216=CARTESIAN_POINT ( 'NONE',  ( -22.67106064244953245, -113.6342314410295842, 5.500000000000000000 ) ) ;
#50218=ORIENTED_EDGE ( 'NONE', *, *, #54519, .F. ) ;
#50229=FACE_OUTER_BOUND ( 'NONE', #51965, .T. ) ;
#50262=CARTESIAN_POINT ( 'NONE',  ( -10.21100092698785033, -95.54625877152835756, -2.500000000000000000 ) ) ;
#50265=VECTOR ( 'NONE', #43824, 1000.000000000000227 ) ;
#50283=ORIENTED_EDGE ( 'NONE', *, *, #13815, .F. ) ;
#50298=ORIENTED_EDGE ( 'NONE', *, *, #40511, .T. ) ;
#50334=DIRECTION ( 'NONE',  ( -0.000000000000000000, -0.000000000000000000, -1.000000000000000000 ) ) ;
#50336=CARTESIAN_POINT ( 'NONE',  ( 10.05638427806949586, -98.76043467366159234, -2.500000000000000000 ) ) ;
#50348=CARTESIAN_POINT ( 'NONE',  ( 22.08297821871651578, -111.8242998470044540, -2.500000000000000000 ) ) ;
#50351=EDGE_CURVE ( 'NONE', #28874, #70060, #71325, .T. ) ;
#50356=CARTESIAN_POINT ( 'NONE',  ( -6.880223345695647197, -142.5202692415819854, 5.500000000000000000 ) ) ;
#50359=CARTESIAN_POINT ( 'NONE',  ( -23.97194136764370498, -131.3950000906648938, 5.500000000000000000 ) ) ;
#50379=DIRECTION ( 'NONE',  ( 0.2306669878475637314, 0.9730327541852493711, 0.000000000000000000 ) ) ;
#50393=ORIENTED_EDGE ( 'NONE', *, *, #60274, .F. ) ;
#50411=ADVANCED_FACE ( 'NONE', ( #20851 ), #60355, .F. ) ;
#50413=DIRECTION ( 'NONE',  ( 0.2867529058022035837, -0.9580045777625452175, 0.000000000000000000 ) ) ;
#50431=PLANE ( 'NONE',  #16346 ) ;
#50484=CARTESIAN_POINT ( 'NONE',  ( 14.59956846177685996, -138.4757300459248484, 5.500000000000000000 ) ) ;
#50509=LINE ( 'NONE', #67058, #17039 ) ;
#50531=LINE ( 'NONE', #20846, #39158 ) ;
#50534=LINE ( 'NONE', #11063, #41820 ) ;
#50545=CARTESIAN_POINT ( 'NONE',  ( -89.17737905728745318, -39.70432723693717492, 5.500000000000000000 ) ) ;
#50558=ORIENTED_EDGE ( 'NONE', *, *, #65354, .F. ) ;
#50560=EDGE_CURVE ( 'NONE', #12079, #1966, #42319, .T. ) ;
#50567=LINE ( 'NONE', #46702, #35758 ) ;
#50590=VECTOR ( 'NONE', #9024, 1000.000000000000000 ) ;
#50594=LINE ( 'NONE', #73148, #25870 ) ;
#50617=VECTOR ( 'NONE', #25203, 1000.000000000000114 ) ;
#50619=CARTESIAN_POINT ( 'NONE',  ( 9.984461079971730157, -95.40710393340120277, 5.500000000000000000 ) ) ;
#50624=CARTESIAN_POINT ( 'NONE',  ( 14.59956846177685996, -138.4757300459248484, 2.500000000000000000 ) ) ;
#50670=DIRECTION ( 'NONE',  ( -0.000000000000000000, -0.000000000000000000, -1.000000000000000000 ) ) ;
#50686=ORIENTED_EDGE ( 'NONE', *, *, #70177, .F. ) ;
#50689=EDGE_CURVE ( 'NONE', #45726, #49118, #26858, .T. ) ;
#50693=EDGE_LOOP ( 'NONE', ( #42181, #27707, #48057, #4554 ) ) ;
#50713=PLANE ( 'NONE',  #20789 ) ;
#50721=DIRECTION ( 'NONE',  ( -0.2306669878475648139, -0.9730327541852491491, 0.000000000000000000 ) ) ;
#50740=DIRECTION ( 'NONE',  ( -0.1850432970638667129, 0.9827303690289281857, 0.000000000000000000 ) ) ;
#50741=ORIENTED_EDGE ( 'NONE', *, *, #52375, .F. ) ;
#50756=EDGE_CURVE ( 'NONE', #61868, #49297, #64057, .T. ) ;
#50800=CARTESIAN_POINT ( 'NONE',  ( 16.84844760790522855, -103.5491698323862124, 5.500000000000000000 ) ) ;
#50822=EDGE_LOOP ( 'NONE', ( #48548, #3362, #49418, #66256 ) ) ;
#50823=EDGE_CURVE ( 'NONE', #44712, #41422, #23095, .T. ) ;
#50852=EDGE_LOOP ( 'NONE', ( #28024, #17686, #29673, #62751 ) ) ;
#50885=DIRECTION ( 'NONE',  ( 0.9730327541852497042, -0.2306669878475623159, 0.000000000000000000 ) ) ;
#50887=ORIENTED_EDGE ( 'NONE', *, *, #73483, .T. ) ;
#50890=CARTESIAN_POINT ( 'NONE',  ( 21.07894319797337701, -103.8699611390234878, -5.500000000000000000 ) ) ;
#50895=DIRECTION ( 'NONE',  ( -0.9997280174009349762, 0.02332147558787671729, 0.000000000000000000 ) ) ;
#50918=DIRECTION ( 'NONE',  ( 0.6691306063588569053, 0.7431448254773954654, 0.000000000000000000 ) ) ;
#50945=DIRECTION ( 'NONE',  ( -0.02332147558787823691, -0.9997280174009349762, 0.000000000000000000 ) ) ;
#50958=VECTOR ( 'NONE', #22244, 1000.000000000000000 ) ;
#50959=LINE ( 'NONE', #22389, #71993 ) ;
#50964=DIRECTION ( 'NONE',  ( -1.000000000000000000, 0.000000000000000000, 0.000000000000000000 ) ) ;
#50985=LINE ( 'NONE', #57371, #40878 ) ;
#51001=DIRECTION ( 'NONE',  ( -0.000000000000000000, -0.000000000000000000, 1.000000000000000000 ) ) ;
#51013=EDGE_CURVE ( 'NONE', #48732, #46548, #26402, .T. ) ;
#51026=ORIENTED_EDGE ( 'NONE', *, *, #37440, .T. ) ;
#51027=ORIENTED_EDGE ( 'NONE', *, *, #47626, .F. ) ;
#51033=ADVANCED_FACE ( 'NONE', ( #38798 ), #62493, .T. ) ;
#51041=DIRECTION ( 'NONE',  ( -0.4796670183876317051, 0.8774505977381971134, 0.000000000000000000 ) ) ;
#51063=VECTOR ( 'NONE', #70974, 1000.000000000000114 ) ;
#51094=CARTESIAN_POINT ( 'NONE',  ( 13.83832728059186046, -142.6495187161941089, 5.500000000000000000 ) ) ;
#51102=EDGE_CURVE ( 'NONE', #29721, #68284, #16603, .T. ) ;
#51141=CARTESIAN_POINT ( 'NONE',  ( 35.50000000000000711, -120.0000000000000000, -2.500000000000000000 ) ) ;
#51168=CARTESIAN_POINT ( 'NONE',  ( -14.87942725330654348, -141.9795960975983178, 5.500000000000000000 ) ) ;
#51193=EDGE_CURVE ( 'NONE', #40320, #64962, #41390, .T. ) ;
#51195=CARTESIAN_POINT ( 'NONE',  ( -18.24502636017239965, -100.7225776329765665, 2.500000000000000000 ) ) ;
#51196=ORIENTED_EDGE ( 'NONE', *, *, #8576, .T. ) ;
#51215=VECTOR ( 'NONE', #44727, 1000.000000000000000 ) ;
#51240=ORIENTED_EDGE ( 'NONE', *, *, #36083, .T. ) ;
#51265=VECTOR ( 'NONE', #14266, 1000.000000000000000 ) ;
#51269=CARTESIAN_POINT ( 'NONE',  ( 103.9230484541331947, -179.9999999999990337, 5.500000000000000000 ) ) ;
#51315=LINE ( 'NONE', #61875, #59545 ) ;
#51326=DIRECTION ( 'NONE',  ( 0.000000000000000000, 0.000000000000000000, -1.000000000000000000 ) ) ;
#51334=LINE ( 'NONE', #57357, #34301 ) ;
#51342=CARTESIAN_POINT ( 'NONE',  ( -23.30023580412278505, -123.4057321492263384, 5.500000000000000000 ) ) ;
#51347=VECTOR ( 'NONE', #26994, 1000.000000000000000 ) ;
#51387=VERTEX_POINT ( 'NONE', #71789 ) ;
#51411=ORIENTED_EDGE ( 'NONE', *, *, #53495, .F. ) ;
#51413=ORIENTED_EDGE ( 'NONE', *, *, #49659, .T. ) ;
#51420=VERTEX_POINT ( 'NONE', #59423 ) ;
#51499=CARTESIAN_POINT ( 'NONE',  ( -23.54415474984308787, -120.4156646670583086, -5.500000000000000000 ) ) ;
#51503=CARTESIAN_POINT ( 'NONE',  ( -21.67772167707813935, -110.8034581014852762, 5.500000000000000000 ) ) ;
#51527=EDGE_LOOP ( 'NONE', ( #16956, #43290, #12315, #27748 ) ) ;
#51541=PLANE ( 'NONE',  #29473 ) ;
#51565=ORIENTED_EDGE ( 'NONE', *, *, #56006, .F. ) ;
#51569=FACE_OUTER_BOUND ( 'NONE', #5736, .T. ) ;
#51600=ORIENTED_EDGE ( 'NONE', *, *, #35635, .F. ) ;
#51624=EDGE_CURVE ( 'NONE', #61202, #31529, #29542, .T. ) ;
#51644=DIRECTION ( 'NONE',  ( 1.000000000000000000, 0.000000000000000000, 0.000000000000000000 ) ) ;
#51649=VECTOR ( 'NONE', #29430, 1000.000000000000000 ) ;
#51652=CARTESIAN_POINT ( 'NONE',  ( -8.826826895187510402, -94.96827758698185562, 5.500000000000000000 ) ) ;
#51660=CARTESIAN_POINT ( 'NONE',  ( 5.822613034544236399, -142.8165987265839760, 5.500000000000000000 ) ) ;
#51703=CARTESIAN_POINT ( 'NONE',  ( 2.117611129180199558, -93.54218975225703048, -5.500000000000000000 ) ) ;
#51766=EDGE_CURVE ( 'NONE', #39841, #10200, #3237, .T. ) ;
#51774=CARTESIAN_POINT ( 'NONE',  ( 16.30584220631899228, -140.9432449716519784, -5.500000000000000000 ) ) ;
#51780=EDGE_LOOP ( 'NONE', ( #27067, #16635, #44877, #62064 ) ) ;
#51801=DIRECTION ( 'NONE',  ( -0.6064928550163511956, -0.7950889364178798102, 0.000000000000000000 ) ) ;
#51803=VECTOR ( 'NONE', #2386, 1000.000000000000000 ) ;
#51855=VECTOR ( 'NONE', #23718, 1000.000000000000114 ) ;
#51910=DIRECTION ( 'NONE',  ( 0.000000000000000000, 0.000000000000000000, 1.000000000000000000 ) ) ;
#51911=CARTESIAN_POINT ( 'NONE',  ( 1.192633404626820770, -120.9097392825245407, 2.500000000000000000 ) ) ;
#51925=DIRECTION ( 'NONE',  ( 0.3311129884571280546, 0.9435911131814402886, 0.000000000000000000 ) ) ;
#51932=CARTESIAN_POINT ( 'NONE',  ( 13.83832728059186046, -142.6495187161941089, 5.500000000000000000 ) ) ;
#51942=ORIENTED_EDGE ( 'NONE', *, *, #37337, .T. ) ;
#51965=EDGE_LOOP ( 'NONE', ( #69877, #63170, #3010, #26806 ) ) ;
#51972=PRODUCT_CONTEXT ( 'NONE', #33027, 'mechanical' ) ;
#51983=ORIENTED_EDGE ( 'NONE', *, *, #29505, .F. ) ;
#51984=DIRECTION ( 'NONE',  ( 0.000000000000000000, 0.000000000000000000, -1.000000000000000000 ) ) ;
#51993=ORIENTED_EDGE ( 'NONE', *, *, #40511, .F. ) ;
#51997=CARTESIAN_POINT ( 'NONE',  ( -10.43921258969510824, -98.89258801967538659, 5.500000000000000000 ) ) ;
#52002=ORIENTED_EDGE ( 'NONE', *, *, #14084, .F. ) ;
#52011=LINE ( 'NONE', #47493, #47728 ) ;
#52015=EDGE_CURVE ( 'NONE', #53859, #47697, #52777, .T. ) ;
#52021=EDGE_LOOP ( 'NONE', ( #7590, #18662, #49913, #14853 ) ) ;
#52035=DIRECTION ( 'NONE',  ( -0.000000000000000000, -0.000000000000000000, -1.000000000000000000 ) ) ;
#52050=DIRECTION ( 'NONE',  ( -0.9580045777625456616, -0.2867529058022021404, 0.000000000000000000 ) ) ;
#52067=VERTEX_POINT ( 'NONE', #18552 ) ;
#52086=LINE ( 'NONE', #11850, #70910 ) ;
#52090=ORIENTED_EDGE ( 'NONE', *, *, #36952, .F. ) ;
#52097=AXIS2_PLACEMENT_3D ( 'NONE', #39418, #51801, #67611 ) ;
#52100=CARTESIAN_POINT ( 'NONE',  ( 23.11608002360578240, -124.4885236261218182, 2.500000000000000000 ) ) ;
#52105=LINE ( 'NONE', #10780, #43287 ) ;
#52106=FACE_OUTER_BOUND ( 'NONE', #59450, .T. ) ;
#52162=VERTEX_POINT ( 'NONE', #71895 ) ;
#52208=ADVANCED_FACE ( 'NONE', ( #20024 ), #3507, .F. ) ;
#52209=DIRECTION ( 'NONE',  ( -0.000000000000000000, -0.000000000000000000, -1.000000000000000000 ) ) ;
#52210=EDGE_CURVE ( 'NONE', #38305, #26020, #3144, .T. ) ;
#52265=DIRECTION ( 'NONE',  ( -0.02332147558787930897, -0.9997280174009348652, 0.000000000000000000 ) ) ;
#52280=EDGE_CURVE ( 'NONE', #7707, #34514, #21882, .T. ) ;
#52287=CARTESIAN_POINT ( 'NONE',  ( -0.1915406271734583221, -121.4877204670710427, 2.500000000000000000 ) ) ;
#52294=FACE_OUTER_BOUND ( 'NONE', #44771, .T. ) ;
#52299=ADVANCED_FACE ( 'NONE', ( #15500, #60992 ), #10981, .F. ) ;
#52304=ORIENTED_EDGE ( 'NONE', *, *, #53986, .T. ) ;
#52318=CARTESIAN_POINT ( 'NONE',  ( -11.59517495878806947, -96.12423995607481686, 5.500000000000000000 ) ) ;
#52336=VECTOR ( 'NONE', #21927, 1000.000000000000000 ) ;
#52367=VECTOR ( 'NONE', #49257, 1000.000000000000114 ) ;
#52375=EDGE_CURVE ( 'NONE', #60419, #23903, #39182, .T. ) ;
#52380=CARTESIAN_POINT ( 'NONE',  ( -7.670864526094549163, -97.73662565058241114, 5.500000000000000000 ) ) ;
#52401=LINE ( 'NONE', #42614, #37890 ) ;
#52413=DIRECTION ( 'NONE',  ( 0.1276937514489679404, 0.9918136447140103451, -0.000000000000000000 ) ) ;
#52439=DIRECTION ( 'NONE',  ( 0.9580045777625456616, 0.2867529058022021404, 0.000000000000000000 ) ) ;
#52441=DIRECTION ( 'NONE',  ( -0.2867529058022035837, 0.9580045777625452175, 0.000000000000000000 ) ) ;
#52445=ORIENTED_EDGE ( 'NONE', *, *, #8147, .F. ) ;
#52459=ORIENTED_EDGE ( 'NONE', *, *, #60635, .T. ) ;
#52475=ADVANCED_FACE ( 'NONE', ( #51569 ), #11337, .F. ) ;
#52484=ORIENTED_EDGE ( 'NONE', *, *, #3402, .T. ) ;
#52504=ORIENTED_EDGE ( 'NONE', *, *, #52210, .T. ) ;
#52552=VERTEX_POINT ( 'NONE', #29000 ) ;
#52555=ADVANCED_FACE ( 'NONE', ( #48152 ), #71063, .F. ) ;
#52584=ORIENTED_EDGE ( 'NONE', *, *, #2957, .F. ) ;
#52591=EDGE_LOOP ( 'NONE', ( #69909, #45942, #61717, #38737 ) ) ;
#52621=VERTEX_POINT ( 'NONE', #2329 ) ;
#52628=ORIENTED_EDGE ( 'NONE', *, *, #29505, .T. ) ;
#52650=FACE_OUTER_BOUND ( 'NONE', #63994, .T. ) ;
#52663=CARTESIAN_POINT ( 'NONE',  ( -3.961125083139900749, -143.2122702051246677, -5.500000000000000000 ) ) ;
#52691=PRODUCT_DEFINITION ( 'UNKNOWN', '', #62881, #72441 ) ;
#52706=ORIENTED_EDGE ( 'NONE', *, *, #43186, .F. ) ;
#52715=ORIENTED_EDGE ( 'NONE', *, *, #6385, .F. ) ;
#52735=DIRECTION ( 'NONE',  ( -0.9580045777625459946, -0.2867529058022011412, 0.000000000000000000 ) ) ;
#52749=VECTOR ( 'NONE', #33746, 1000.000000000000000 ) ;
#52777=LINE ( 'NONE', #210, #29259 ) ;
#52794=VECTOR ( 'NONE', #21186, 1000.000000000000227 ) ;
#52797=VERTEX_POINT ( 'NONE', #49982 ) ;
#52814=CARTESIAN_POINT ( 'NONE',  ( 26.47460221209471598, -121.8961639463267090, -5.500000000000000000 ) ) ;
#52820=ORIENTED_EDGE ( 'NONE', *, *, #43218, .F. ) ;
#52850=VECTOR ( 'NONE', #45628, 1000.000000000000114 ) ;
#52864=CARTESIAN_POINT ( 'NONE',  ( 19.29194287201271862, -133.5026271600380880, 5.500000000000000000 ) ) ;
#52870=EDGE_CURVE ( 'NONE', #27007, #44712, #55267, .T. ) ;
#52894=EDGE_LOOP ( 'NONE', ( #2634, #68350, #36402, #4557 ) ) ;
#52911=ORIENTED_EDGE ( 'NONE', *, *, #11159, .T. ) ;
#52925=DIRECTION ( 'NONE',  ( -0.000000000000000000, -0.000000000000000000, -1.000000000000000000 ) ) ;
#53014=CARTESIAN_POINT ( 'NONE',  ( -21.33958957442910886, -129.9559990355020034, 5.500000000000000000 ) ) ;
#53026=CARTESIAN_POINT ( 'NONE',  ( -23.97194136764370498, -131.3950000906648938, -5.500000000000000000 ) ) ;
#53027=PLANE ( 'NONE',  #59061 ) ;
#53033=LINE ( 'NONE', #13538, #18743 ) ;
#53084=VERTEX_POINT ( 'NONE', #73909 ) ;
#53108=CARTESIAN_POINT ( 'NONE',  ( 23.11608002360578240, -124.4885236261218182, -5.500000000000000000 ) ) ;
#53113=CARTESIAN_POINT ( 'NONE',  ( -17.26469406256017791, -140.1601175325492648, 5.500000000000000000 ) ) ;
#53156=EDGE_LOOP ( 'NONE', ( #52445, #59658, #60397, #1381 ) ) ;
#53161=EDGE_CURVE ( 'NONE', #42454, #27599, #38599, .T. ) ;
#53171=FACE_OUTER_BOUND ( 'NONE', #47368, .T. ) ;
#53219=CARTESIAN_POINT ( 'NONE',  ( -32.50000000000000000, -120.0000000000000000, -2.500000000000000000 ) ) ;
#53222=CARTESIAN_POINT ( 'NONE',  ( 8.700667342345820288, -98.11853780484867116, 5.500000000000000000 ) ) ;
#53234=CARTESIAN_POINT ( 'NONE',  ( 12.50000000000000000, -132.5000000000000000, 2.500000000000000000 ) ) ;
#53254=PLANE ( 'NONE',  #34030 ) ;
#53291=ADVANCED_FACE ( 'NONE', ( #12641 ), #69788, .F. ) ;
#53293=VECTOR ( 'NONE', #26861, 1000.000000000000000 ) ;
#53304=DIRECTION ( 'NONE',  ( 0.4796670183876317051, -0.8774505977381971134, 0.000000000000000000 ) ) ;
#53310=LINE ( 'NONE', #36375, #21980 ) ;
#53316=EDGE_CURVE ( 'NONE', #19317, #28874, #69065, .T. ) ;
#53319=VECTOR ( 'NONE', #40750, 1000.000000000000000 ) ;
#53327=ADVANCED_FACE ( 'NONE', ( #17550 ), #13008, .T. ) ;
#53344=ORIENTED_EDGE ( 'NONE', *, *, #37887, .F. ) ;
#53356=AXIS2_PLACEMENT_3D ( 'NONE', #58529, #41994, #64930 ) ;
#53365=ORIENTED_EDGE ( 'NONE', *, *, #73483, .F. ) ;
#53369=EDGE_LOOP ( 'NONE', ( #41510, #6407, #63699, #13401 ) ) ;
#53388=PLANE ( 'NONE',  #48845 ) ;
#53407=CARTESIAN_POINT ( 'NONE',  ( -15.44521549751111422, -137.7748507232956001, 5.500000000000000000 ) ) ;
#53417=LINE ( 'NONE', #63972, #46744 ) ;
#53443=DIRECTION ( 'NONE',  ( 0.2867529058022035837, -0.9580045777625452175, 0.000000000000000000 ) ) ;
#53460=ADVANCED_FACE ( 'NONE', ( #20784 ), #43738, .F. ) ;
#53462=CARTESIAN_POINT ( 'NONE',  ( 23.30762065077924916, -123.0008031590507329, -2.500000000000000000 ) ) ;
#53467=ORIENTED_EDGE ( 'NONE', *, *, #50823, .T. ) ;
#53473=VECTOR ( 'NONE', #41192, 1000.000000000000000 ) ;
#53479=ADVANCED_FACE ( 'NONE', ( #38078 ), #44474, .F. ) ;
#53495=EDGE_CURVE ( 'NONE', #31458, #23125, #67390, .T. ) ;
#53502=DIRECTION ( 'NONE',  ( -0.8225049752423791993, -0.5687579148473745905, 0.000000000000000000 ) ) ;
#53539=ORIENTED_EDGE ( 'NONE', *, *, #27471, .T. ) ;
#53545=LINE ( 'NONE', #2084, #60736 ) ;
#53565=ORIENTED_EDGE ( 'NONE', *, *, #17000, .F. ) ;
#53584=DIRECTION ( 'NONE',  ( -0.2867529058022035837, 0.9580045777625452175, 0.000000000000000000 ) ) ;
#53585=DIRECTION ( 'NONE',  ( -0.8774505977381971134, -0.4796670183876317051, 0.000000000000000000 ) ) ;
#53588=CARTESIAN_POINT ( 'NONE',  ( 19.29194287201271862, -133.5026271600380880, 5.500000000000000000 ) ) ;
#53617=DIRECTION ( 'NONE',  ( -0.6862798483830544471, -0.7273375899149802093, 0.000000000000000000 ) ) ;
#53703=PLANE ( 'NONE',  #15226 ) ;
#53710=ORIENTED_EDGE ( 'NONE', *, *, #43186, .T. ) ;
#53722=LINE ( 'NONE', #2641, #11676 ) ;
#53726=EDGE_CURVE ( 'NONE', #44676, #105, #34286, .T. ) ;
#53727=VECTOR ( 'NONE', #19073, 1000.000000000000000 ) ;
#53740=CARTESIAN_POINT ( 'NONE',  ( 21.85433023846371370, -135.0628101570779620, 5.500000000000000000 ) ) ;
#53751=EDGE_CURVE ( 'NONE', #43669, #71014, #23027, .T. ) ;
#53759=VECTOR ( 'NONE', #46531, 999.9999999999998863 ) ;
#53761=LINE ( 'NONE', #25198, #29106 ) ;
#53790=CARTESIAN_POINT ( 'NONE',  ( 20.10151712711562766, -102.7321394148470830, -2.500000000000000000 ) ) ;
#53802=ORIENTED_EDGE ( 'NONE', *, *, #6525, .T. ) ;
#53808=CARTESIAN_POINT ( 'NONE',  ( 25.38712131070745315, -112.4010479962415872, -2.500000000000000000 ) ) ;
#53846=DIRECTION ( 'NONE',  ( -0.000000000000000000, -0.000000000000000000, -1.000000000000000000 ) ) ;
#53859=VERTEX_POINT ( 'NONE', #63985 ) ;
#53866=CARTESIAN_POINT ( 'NONE',  ( 22.94323693612312809, -114.6983135802921083, 5.500000000000000000 ) ) ;
#53883=EDGE_CURVE ( 'NONE', #27833, #38563, #69344, .T. ) ;
#53885=CARTESIAN_POINT ( 'NONE',  ( -6.880223345695647197, -142.5202692415819854, 2.500000000000000000 ) ) ;
#53894=CARTESIAN_POINT ( 'NONE',  ( 2.874421927457452952, -143.3717286177755739, 5.500000000000000000 ) ) ;
#53898=EDGE_CURVE ( 'NONE', #28347, #39126, #13308, .T. ) ;
#53925=CARTESIAN_POINT ( 'NONE',  ( -21.33958957442910886, -129.9559990355020034, 5.500000000000000000 ) ) ;
#53946=CARTESIAN_POINT ( 'NONE',  ( -13.05994868825747446, -139.5943292883446532, 5.500000000000000000 ) ) ;
#53950=ORIENTED_EDGE ( 'NONE', *, *, #54236, .F. ) ;
#53952=VECTOR ( 'NONE', #25995, 1000.000000000000000 ) ;
#53975=DIRECTION ( 'NONE',  ( 0.5200609990133008287, 0.8541291221503266584, -0.000000000000000000 ) ) ;
#53986=EDGE_CURVE ( 'NONE', #58705, #2902, #71557, .T. ) ;
#53992=ORIENTED_EDGE ( 'NONE', *, *, #10696, .F. ) ;
#54001=DIRECTION ( 'NONE',  ( -0.5200609990132993854, -0.8541291221503274356, 0.000000000000000000 ) ) ;
#54009=AXIS2_PLACEMENT_3D ( 'NONE', #24548, #23086, #51644 ) ;
#54010=ORIENTED_EDGE ( 'NONE', *, *, #303, .F. ) ;
#54028=LINE ( 'NONE', #13782, #73426 ) ;
#54032=ORIENTED_EDGE ( 'NONE', *, *, #55945, .T. ) ;
#54047=VERTEX_POINT ( 'NONE', #43006 ) ;
#54053=CARTESIAN_POINT ( 'NONE',  ( -0.1915406271734583221, -121.4877204670710427, -2.500000000000000000 ) ) ;
#54054=DIRECTION ( 'NONE',  ( -0.8541291221503261033, 0.5200609990133016058, 0.000000000000000000 ) ) ;
#54060=DIRECTION ( 'NONE',  ( -0.000000000000000000, -0.000000000000000000, -1.000000000000000000 ) ) ;
#54086=ADVANCED_FACE ( 'NONE', ( #73777 ), #21160, .T. ) ;
#54089=VERTEX_POINT ( 'NONE', #39216 ) ;
#54096=CARTESIAN_POINT ( 'NONE',  ( -19.27444613274700913, -101.8135840178490668, 2.500000000000000000 ) ) ;
#54118=EDGE_LOOP ( 'NONE', ( #41988, #69900, #55016, #54360 ) ) ;
#54119=DIRECTION ( 'NONE',  ( 1.000000000000000000, 0.000000000000000000, -0.000000000000000000 ) ) ;
#54121=VERTEX_POINT ( 'NONE', #15533 ) ;
#54129=LINE ( 'NONE', #69919, #35865 ) ;
#54135=DIRECTION ( 'NONE',  ( -0.8090169943749504489, 0.5877852522924689183, 0.000000000000000000 ) ) ;
#54155=EDGE_CURVE ( 'NONE', #44097, #6594, #67405, .T. ) ;
#54158=LINE ( 'NONE', #2689, #15464 ) ;
#54189=VECTOR ( 'NONE', #65687, 1000.000000000000114 ) ;
#54203=ORIENTED_EDGE ( 'NONE', *, *, #54804, .T. ) ;
#54210=ORIENTED_EDGE ( 'NONE', *, *, #49036, .T. ) ;
#54211=CARTESIAN_POINT ( 'NONE',  ( -21.67772167707813935, -110.8034581014852762, 5.500000000000000000 ) ) ;
#54222=LINE ( 'NONE', #47103, #14336 ) ;
#54233=ORIENTED_EDGE ( 'NONE', *, *, #42681, .T. ) ;
#54236=EDGE_CURVE ( 'NONE', #27007, #31458, #71003, .T. ) ;
#54244=ORIENTED_EDGE ( 'NONE', *, *, #46000, .F. ) ;
#54257=EDGE_CURVE ( 'NONE', #4558, #30043, #53722, .T. ) ;
#54259=CARTESIAN_POINT ( 'NONE',  ( 9.984461079971730157, -95.40710393340121698, -2.500000000000000000 ) ) ;
#54270=CARTESIAN_POINT ( 'NONE',  ( -0.9774260708577104939, -118.8621782758236378, -2.500000000000000000 ) ) ;
#54274=EDGE_LOOP ( 'NONE', ( #40218, #67065, #27637, #73914 ) ) ;
#54275=VECTOR ( 'NONE', #68002, 1000.000000000000000 ) ;
#54292=CARTESIAN_POINT ( 'NONE',  ( 9.984461079971730157, -95.40710393340120277, -5.500000000000000000 ) ) ;
#54333=DIRECTION ( 'NONE',  ( 0.9730327541852497042, -0.2306669878475622604, 0.000000000000000000 ) ) ;
#54340=VECTOR ( 'NONE', #49772, 999.9999999999998863 ) ;
#54346=CYLINDRICAL_SURFACE ( 'NONE', #73378, 30.50000000000000000 ) ;
#54360=ORIENTED_EDGE ( 'NONE', *, *, #73188, .T. ) ;
#54383=CARTESIAN_POINT ( 'NONE',  ( 25.81725066941077529, -113.8380548628854854, 5.500000000000000000 ) ) ;
#54384=ORIENTED_EDGE ( 'NONE', *, *, #44482, .F. ) ;
#54427=EDGE_CURVE ( 'NONE', #71014, #67963, #55580, .T. ) ;
#54446=DIRECTION ( 'NONE',  ( -1.000000000000000000, 0.000000000000000000, 0.000000000000000000 ) ) ;
#54448=FACE_OUTER_BOUND ( 'NONE', #62347, .T. ) ;
#54453=ORIENTED_EDGE ( 'NONE', *, *, #47393, .T. ) ;
#54463=VECTOR ( 'NONE', #8477, 1000.000000000000114 ) ;
#54465=ORIENTED_EDGE ( 'NONE', *, *, #5274, .T. ) ;
#54471=FACE_OUTER_BOUND ( 'NONE', #19378, .T. ) ;
#54473=DIRECTION ( 'NONE',  ( 0.6691306063588569053, 0.7431448254773954654, 0.000000000000000000 ) ) ;
#54477=EDGE_CURVE ( 'NONE', #26154, #8157, #32260, .T. ) ;
#54495=DIRECTION ( 'NONE',  ( 0.000000000000000000, 0.000000000000000000, 1.000000000000000000 ) ) ;
#54503=DIRECTION ( 'NONE',  ( -0.02332147558787930897, -0.9997280174009348652, 0.000000000000000000 ) ) ;
#54507=DIRECTION ( 'NONE',  ( 0.7585478161175716050, 0.6516173805718067369, 0.000000000000000000 ) ) ;
#54511=CARTESIAN_POINT ( 'NONE',  ( 5.822613034544236399, -142.8165987265839760, -5.500000000000000000 ) ) ;
#54517=CARTESIAN_POINT ( 'NONE',  ( -9.055038557894883766, -98.31460683512894150, -2.500000000000000000 ) ) ;
#54519=EDGE_CURVE ( 'NONE', #61799, #70823, #44688, .T. ) ;
#54520=CARTESIAN_POINT ( 'NONE',  ( -22.53294031248082163, -134.0273518838794757, 5.500000000000000000 ) ) ;
#54528=DIRECTION ( 'NONE',  ( 0.3311129884571281101, 0.9435911131814402886, 0.000000000000000000 ) ) ;
#54537=AXIS2_PLACEMENT_3D ( 'NONE', #7561, #59810, #54528 ) ;
#54541=AXIS2_PLACEMENT_3D ( 'NONE', #18990, #1018, #46106 ) ;
#54542=CARTESIAN_POINT ( 'NONE',  ( 0.000000000000000000, -120.0000000000000000, 2.500000000000000000 ) ) ;
#54551=LINE ( 'NONE', #24501, #10422 ) ;
#54555=EDGE_CURVE ( 'NONE', #68902, #46309, #11932, .T. ) ;
#54584=CARTESIAN_POINT ( 'NONE',  ( -26.53422223201112828, -120.6595836127786043, 5.500000000000000000 ) ) ;
#54620=DIRECTION ( 'NONE',  ( 0.000000000000000000, 0.000000000000000000, 1.000000000000000000 ) ) ;
#54630=EDGE_LOOP ( 'NONE', ( #70603, #2762, #51196, #52459 ) ) ;
#54633=VECTOR ( 'NONE', #14516, 1000.000000000000227 ) ;
#54688=DIRECTION ( 'NONE',  ( -0.9966891607226786576, -0.08130631524009861166, 0.000000000000000000 ) ) ;
#54711=VECTOR ( 'NONE', #65579, 1000.000000000000114 ) ;
#54724=AXIS2_PLACEMENT_3D ( 'NONE', #20419, #21138, #49351 ) ;
#54765=ORIENTED_EDGE ( 'NONE', *, *, #15779, .T. ) ;
#54804=EDGE_CURVE ( 'NONE', #73248, #43631, #60772, .T. ) ;
#54808=AXIS2_PLACEMENT_3D ( 'NONE', #57995, #6139, #40709 ) ;
#54812=EDGE_CURVE ( 'NONE', #52552, #57541, #25805, .T. ) ;
#54821=EDGE_CURVE ( 'NONE', #64729, #20698, #37477, .T. ) ;
#54837=ORIENTED_EDGE ( 'NONE', *, *, #68016, .T. ) ;
#54845=FACE_BOUND ( 'NONE', #38654, .T. ) ;
#54846=EDGE_CURVE ( 'NONE', #15838, #41508, #67142, .T. ) ;
#54850=ORIENTED_EDGE ( 'NONE', *, *, #25570, .F. ) ;
#54859=ORIENTED_EDGE ( 'NONE', *, *, #55741, .T. ) ;
#54866=PLANE ( 'NONE',  #42802 ) ;
#54896=EDGE_CURVE ( 'NONE', #73780, #7680, #2561, .T. ) ;
#54904=AXIS2_PLACEMENT_3D ( 'NONE', #15810, #62812, #22948 ) ;
#54914=VERTEX_POINT ( 'NONE', #14146 ) ;
#54927=ORIENTED_EDGE ( 'NONE', *, *, #7892, .F. ) ;
#54939=DIRECTION ( 'NONE',  ( 0.7273375899149812085, -0.6862798483830533369, 0.000000000000000000 ) ) ;
#54944=ORIENTED_EDGE ( 'NONE', *, *, #8201, .T. ) ;
#54955=ORIENTED_EDGE ( 'NONE', *, *, #40770, .T. ) ;
#54962=AXIS2_PLACEMENT_3D ( 'NONE', #15333, #61220, #51041 ) ;
#54984=VECTOR ( 'NONE', #39790, 1000.000000000000114 ) ;
#54993=LINE ( 'NONE', #21509, #20772 ) ;
#54995=ORIENTED_EDGE ( 'NONE', *, *, #16116, .F. ) ;
#55006=VERTEX_POINT ( 'NONE', #62258 ) ;
#55009=AXIS2_PLACEMENT_3D ( 'NONE', #61873, #72749, #49827 ) ;
#55016=ORIENTED_EDGE ( 'NONE', *, *, #57213, .F. ) ;
#55019=EDGE_CURVE ( 'NONE', #42393, #23530, #31471, .T. ) ;
#55037=PLANE ( 'NONE',  #58303 ) ;
#55052=CARTESIAN_POINT ( 'NONE',  ( -7.670864526094549163, -97.73662565058241114, -5.500000000000000000 ) ) ;
#55053=DIRECTION ( 'NONE',  ( 0.7585478161175706058, 0.6516173805718080692, -0.000000000000000000 ) ) ;
#55054=VECTOR ( 'NONE', #27803, 1000.000000000000000 ) ;
#55103=VERTEX_POINT ( 'NONE', #12588 ) ;
#55116=VERTEX_POINT ( 'NONE', #1722 ) ;
#55123=DIRECTION ( 'NONE',  ( 0.7273375899149802093, -0.6862798483830544471, 0.000000000000000000 ) ) ;
#55129=FACE_OUTER_BOUND ( 'NONE', #28557, .T. ) ;
#55137=LINE ( 'NONE', #5048, #27782 ) ;
#55143=VERTEX_POINT ( 'NONE', #24610 ) ;
#55182=ORIENTED_EDGE ( 'NONE', *, *, #57321, .T. ) ;
#55196=DIRECTION ( 'NONE',  ( -0.000000000000000000, -0.000000000000000000, -1.000000000000000000 ) ) ;
#55230=CARTESIAN_POINT ( 'NONE',  ( -5.420674214417706693, -142.8662697233533265, -2.500000000000000000 ) ) ;
#55233=EDGE_CURVE ( 'NONE', #1704, #6231, #58831, .T. ) ;
#55267=LINE ( 'NONE', #62033, #59428 ) ;
#55278=ORIENTED_EDGE ( 'NONE', *, *, #58382, .T. ) ;
#55301=ORIENTED_EDGE ( 'NONE', *, *, #38622, .F. ) ;
#55309=EDGE_LOOP ( 'NONE', ( #33135, #39011, #35335, #60483 ) ) ;
#55311=FACE_OUTER_BOUND ( 'NONE', #74326, .T. ) ;
#55322=EDGE_CURVE ( 'NONE', #11947, #9134, #47119, .T. ) ;
#55324=CARTESIAN_POINT ( 'NONE',  ( -18.12185313557660038, -104.9634299478706794, -5.500000000000000000 ) ) ;
#55325=DIRECTION ( 'NONE',  ( -0.000000000000000000, -0.000000000000000000, -1.000000000000000000 ) ) ;
#55331=CARTESIAN_POINT ( 'NONE',  ( -15.44521549751111422, -137.7748507232956001, -5.500000000000000000 ) ) ;
#55353=ORIENTED_EDGE ( 'NONE', *, *, #19699, .T. ) ;
#55354=CARTESIAN_POINT ( 'NONE',  ( -0.7195005275814509993, -118.6838241033926948, -2.500000000000000000 ) ) ;
#55359=EDGE_CURVE ( 'NONE', #12142, #38305, #7261, .T. ) ;
#55379=DIRECTION ( 'NONE',  ( 0.4279312458752976833, 0.9038112904824853189, -0.000000000000000000 ) ) ;
#55419=VECTOR ( 'NONE', #17214, 1000.000000000000000 ) ;
#55426=LINE ( 'NONE', #22329, #50176 ) ;
#55460=AXIS2_PLACEMENT_3D ( 'NONE', #6242, #64479, #52441 ) ;
#55469=VERTEX_POINT ( 'NONE', #55331 ) ;
#55470=ORIENTED_EDGE ( 'NONE', *, *, #29854, .F. ) ;
#55536=EDGE_CURVE ( 'NONE', #64729, #70242, #45922, .T. ) ;
#55580=LINE ( 'NONE', #66133, #3339 ) ;
#55591=CARTESIAN_POINT ( 'NONE',  ( -0.8815729230226007074, -93.47222532549339746, -2.500000000000000000 ) ) ;
#55607=DIRECTION ( 'NONE',  ( 0.3311129884571304971, 0.9435911131814395114, -0.000000000000000000 ) ) ;
#55614=PLANE ( 'NONE',  #44568 ) ;
#55617=EDGE_CURVE ( 'NONE', #29007, #68795, #28979, .T. ) ;
#55640=DIRECTION ( 'NONE',  ( -0.000000000000000000, -0.000000000000000000, 1.000000000000000000 ) ) ;
#55655=ORIENTED_EDGE ( 'NONE', *, *, #70177, .T. ) ;
#55681=DIRECTION ( 'NONE',  ( -0.9966891607226786576, -0.08130631524009861166, 0.000000000000000000 ) ) ;
#55697=DIRECTION ( 'NONE',  ( 0.4279312458752991266, 0.9038112904824847638, 0.000000000000000000 ) ) ;
#55698=LINE ( 'NONE', #55324, #36684 ) ;
#55714=AXIS2_PLACEMENT_3D ( 'NONE', #51503, #59, #34579 ) ;
#55734=CARTESIAN_POINT ( 'NONE',  ( 12.13205353604972814, -140.1820037904669789, -2.500000000000000000 ) ) ;
#55741=EDGE_CURVE ( 'NONE', #71076, #48732, #53761, .T. ) ;
#55780=ORIENTED_EDGE ( 'NONE', *, *, #73732, .F. ) ;
#55807=VECTOR ( 'NONE', #33381, 1000.000000000000114 ) ;
#55809=CARTESIAN_POINT ( 'NONE',  ( -13.05994868825747446, -139.5943292883446532, 5.500000000000000000 ) ) ;
#55828=CARTESIAN_POINT ( 'NONE',  ( -26.53422223201112828, -120.6595836127786043, -5.500000000000000000 ) ) ;
#55832=ORIENTED_EDGE ( 'NONE', *, *, #55019, .T. ) ;
#55847=DIRECTION ( 'NONE',  ( -0.000000000000000000, -0.000000000000000000, -1.000000000000000000 ) ) ;
#55883=EDGE_LOOP ( 'NONE', ( #14218, #42479, #26690, #7020 ) ) ;
#55884=ORIENTED_EDGE ( 'NONE', *, *, #46000, .T. ) ;
#55894=PLANE ( 'NONE',  #47520 ) ;
#55916=DIRECTION ( 'NONE',  ( -0.000000000000000000, -0.000000000000000000, -1.000000000000000000 ) ) ;
#55919=EDGE_CURVE ( 'NONE', #64962, #7487, #20663, .T. ) ;
#55938=PLANE ( 'NONE',  #63409 ) ;
#55945=EDGE_CURVE ( 'NONE', #49062, #40306, #20281, .T. ) ;
#55947=CARTESIAN_POINT ( 'NONE',  ( -19.90058851926621841, -132.5883508287165853, -2.500000000000000000 ) ) ;
#55973=ORIENTED_EDGE ( 'NONE', *, *, #45950, .T. ) ;
#55974=CARTESIAN_POINT ( 'NONE',  ( 25.38712131070745315, -112.4010479962415872, 2.500000000000000000 ) ) ;
#55979=LINE ( 'NONE', #62006, #21701 ) ;
#56006=EDGE_CURVE ( 'NONE', #19127, #16009, #32751, .T. ) ;
#56020=ORIENTED_EDGE ( 'NONE', *, *, #19501, .F. ) ;
#56026=DIRECTION ( 'NONE',  ( -0.6516173805718079581, 0.7585478161175704948, 0.000000000000000000 ) ) ;
#56027=ORIENTED_EDGE ( 'NONE', *, *, #49134, .T. ) ;
#56042=VERTEX_POINT ( 'NONE', #16889 ) ;
#56079=DIRECTION ( 'NONE',  ( -0.3311129884571281101, -0.9435911131814402886, 0.000000000000000000 ) ) ;
#56092=APPLICATION_CONTEXT ( 'automotive_design' ) ;
#56099=ORIENTED_EDGE ( 'NONE', *, *, #6385, .T. ) ;
#56102=CARTESIAN_POINT ( 'NONE',  ( -16.06301359042743115, -102.7814171781257357, -2.500000000000000000 ) ) ;
#56104=VECTOR ( 'NONE', #15209, 1000.000000000000000 ) ;
#56114=CARTESIAN_POINT ( 'NONE',  ( 23.41451323550360186, -132.5004227906269989, 5.500000000000000000 ) ) ;
#56123=PLANE ( 'NONE',  #37156 ) ;
#56124=ADVANCED_FACE ( 'NONE', ( #63499 ), #50713, .F. ) ;
#56126=EDGE_CURVE ( 'NONE', #68048, #44533, #68014, .T. ) ;
#56133=ORIENTED_EDGE ( 'NONE', *, *, #28608, .F. ) ;
#56157=DIRECTION ( 'NONE',  ( 0.6516173805718079581, -0.7585478161175704948, 0.000000000000000000 ) ) ;
#56172=ORIENTED_EDGE ( 'NONE', *, *, #72023, .F. ) ;
#56209=EDGE_CURVE ( 'NONE', #38913, #8717, #53310, .T. ) ;
#56211=ORIENTED_EDGE ( 'NONE', *, *, #43558, .T. ) ;
#56226=ORIENTED_EDGE ( 'NONE', *, *, #17389, .T. ) ;
#56230=LINE ( 'NONE', #24604, #62687 ) ;
#56254=CARTESIAN_POINT ( 'NONE',  ( -23.42219527698293646, -121.9106984081423803, 2.500000000000000000 ) ) ;
#56297=LINE ( 'NONE', #27715, #47474 ) ;
#56309=LINE ( 'NONE', #15710, #66458 ) ;
#56311=VECTOR ( 'NONE', #12201, 1000.000000000000000 ) ;
#56351=VECTOR ( 'NONE', #30399, 1000.000000000000000 ) ;
#56365=FACE_OUTER_BOUND ( 'NONE', #14584, .T. ) ;
#56370=CARTESIAN_POINT ( 'NONE',  ( -1.029419772574582836, -121.0910063848724718, -2.500000000000000000 ) ) ;
#56380=VECTOR ( 'NONE', #49722, 1000.000000000000000 ) ;
#56385=DIRECTION ( 'NONE',  ( -0.000000000000000000, -0.000000000000000000, -1.000000000000000000 ) ) ;
#56397=ADVANCED_FACE ( 'NONE', ( #16422 ), #22436, .F. ) ;
#56441=ORIENTED_EDGE ( 'NONE', *, *, #53883, .T. ) ;
#56458=EDGE_CURVE ( 'NONE', #46172, #19845, #62296, .T. ) ;
#56479=EDGE_CURVE ( 'NONE', #45901, #43278, #34077, .T. ) ;
#56497=ORIENTED_EDGE ( 'NONE', *, *, #37440, .F. ) ;
#56547=DIRECTION ( 'NONE',  ( -0.7950889364178796992, 0.6064928550163510845, 0.000000000000000000 ) ) ;
#56549=CARTESIAN_POINT ( 'NONE',  ( -26.53422223201112828, -120.6595836127786043, -5.500000000000000000 ) ) ;
#56556=CARTESIAN_POINT ( 'NONE',  ( -16.06301359042743115, -102.7814171781257357, 5.500000000000000000 ) ) ;
#56565=DIRECTION ( 'NONE',  ( 0.9435911131814395114, -0.3311129884571304971, 0.000000000000000000 ) ) ;
#56574=ADVANCED_FACE ( 'NONE', ( #6980 ), #47216, .F. ) ;
#56603=DIRECTION ( 'NONE',  ( -0.9997280174009349762, 0.02332147558787823691, 0.000000000000000000 ) ) ;
#56640=ORIENTED_EDGE ( 'NONE', *, *, #565, .F. ) ;
#56666=CARTESIAN_POINT ( 'NONE',  ( -11.59517495878806947, -96.12423995607481686, 5.500000000000000000 ) ) ;
#56667=DIRECTION ( 'NONE',  ( 0.8541291221503261033, -0.5200609990133016058, 0.000000000000000000 ) ) ;
#56680=DIRECTION ( 'NONE',  ( -0.2306669878475637314, -0.9730327541852493711, 0.000000000000000000 ) ) ;
#56693=VERTEX_POINT ( 'NONE', #16598 ) ;
#56725=ORIENTED_EDGE ( 'NONE', *, *, #38096, .F. ) ;
#56744=EDGE_CURVE ( 'NONE', #22108, #63004, #21869, .T. ) ;
#56747=DIRECTION ( 'NONE',  ( -0.9038112904824853189, 0.4279312458752976833, 0.000000000000000000 ) ) ;
#56773=PLANE ( 'NONE',  #43998 ) ;
#56777=EDGE_LOOP ( 'NONE', ( #59528, #20795, #31290, #6217 ) ) ;
#56786=VERTEX_POINT ( 'NONE', #32027 ) ;
#56791=CARTESIAN_POINT ( 'NONE',  ( 11.34017801569539685, -96.04900080221412395, 2.500000000000000000 ) ) ;
#56797=EDGE_LOOP ( 'NONE', ( #45961, #41771 ) ) ;
#56811=LINE ( 'NONE', #809, #47898 ) ;
#56817=VECTOR ( 'NONE', #12161, 1000.000000000000000 ) ;
#56886=VERTEX_POINT ( 'NONE', #12071 ) ;
#56942=CARTESIAN_POINT ( 'NONE',  ( 16.30584220631899228, -140.9432449716519784, 5.500000000000000000 ) ) ;
#56952=VECTOR ( 'NONE', #16407, 1000.000000000000000 ) ;
#56961=VERTEX_POINT ( 'NONE', #35010 ) ;
#56963=ORIENTED_EDGE ( 'NONE', *, *, #37207, .F. ) ;
#56977=CARTESIAN_POINT ( 'NONE',  ( -11.59517495878806947, -96.12423995607481686, 5.500000000000000000 ) ) ;
#56994=ORIENTED_EDGE ( 'NONE', *, *, #3592, .T. ) ;
#57011=CARTESIAN_POINT ( 'NONE',  ( 23.49916127795269460, -121.5130826919798039, 2.500000000000000000 ) ) ;
#57021=DIRECTION ( 'NONE',  ( -0.000000000000000000, -0.000000000000000000, -1.000000000000000000 ) ) ;
#57022=DIRECTION ( 'NONE',  ( -0.9580045777625452175, -0.2867529058022035837, 0.000000000000000000 ) ) ;
#57023=DIRECTION ( 'NONE',  ( 0.8541291221503275466, -0.5200609990132993854, 0.000000000000000000 ) ) ;
#57039=ORIENTED_EDGE ( 'NONE', *, *, #16116, .T. ) ;
#57050=ORIENTED_EDGE ( 'NONE', *, *, #68771, .T. ) ;
#57062=CARTESIAN_POINT ( 'NONE',  ( 12.50000000000000000, -132.5000000000000000, 2.500000000000000000 ) ) ;
#57065=FACE_OUTER_BOUND ( 'NONE', #9965, .T. ) ;
#57096=ORIENTED_EDGE ( 'NONE', *, *, #57302, .F. ) ;
#57114=LINE ( 'NONE', #58574, #63686 ) ;
#57154=ADVANCED_FACE ( 'NONE', ( #36111 ), #7546, .F. ) ;
#57158=CARTESIAN_POINT ( 'NONE',  ( 0.000000000000000000, -120.0000000000000000, 2.500000000000000000 ) ) ;
#57163=CARTESIAN_POINT ( 'NONE',  ( -7.572224309238338336, -145.4393675041377492, 5.500000000000000000 ) ) ;
#57174=ORIENTED_EDGE ( 'NONE', *, *, #23402, .F. ) ;
#57201=ORIENTED_EDGE ( 'NONE', *, *, #51193, .F. ) ;
#57213=EDGE_CURVE ( 'NONE', #46917, #11307, #71786, .T. ) ;
#57223=CARTESIAN_POINT ( 'NONE',  ( -0.4966694826856976608, -121.4153866697721611, 2.500000000000000000 ) ) ;
#57244=ORIENTED_EDGE ( 'NONE', *, *, #65178, .T. ) ;
#57253=ORIENTED_EDGE ( 'NONE', *, *, #2321, .F. ) ;
#57257=VECTOR ( 'NONE', #41595, 1000.000000000000000 ) ;
#57265=ORIENTED_EDGE ( 'NONE', *, *, #4169, .T. ) ;
#57302=EDGE_CURVE ( 'NONE', #2654, #58705, #67280, .T. ) ;
#57321=EDGE_CURVE ( 'NONE', #38563, #40323, #28907, .T. ) ;
#57344=DIRECTION ( 'NONE',  ( -0.4796670183876317051, 0.8774505977381972244, 0.000000000000000000 ) ) ;
#57357=CARTESIAN_POINT ( 'NONE',  ( -0.9515373497862389396, -96.47140937769621871, 5.500000000000000000 ) ) ;
#57371=CARTESIAN_POINT ( 'NONE',  ( -0.9515373497862389396, -96.47140937769621871, 5.500000000000000000 ) ) ;
#57380=LINE ( 'NONE', #57756, #61107 ) ;
#57386=DIRECTION ( 'NONE',  ( -0.9435911131814398445, 0.3311129884571295534, 0.000000000000000000 ) ) ;
#57390=VECTOR ( 'NONE', #69170, 1000.000000000000000 ) ;
#57490=AXIS2_PLACEMENT_3D ( 'NONE', #67774, #33545, #33922 ) ;
#57491=LINE ( 'NONE', #29270, #41672 ) ;
#57511=DIRECTION ( 'NONE',  ( 0.000000000000000000, 0.000000000000000000, 1.000000000000000000 ) ) ;
#57517=PLANE ( 'NONE',  #73112 ) ;
#57519=EDGE_LOOP ( 'NONE', ( #63764, #10151, #56027, #65088 ) ) ;
#57541=VERTEX_POINT ( 'NONE', #5083 ) ;
#57544=VERTEX_POINT ( 'NONE', #33625 ) ;
#57588=VECTOR ( 'NONE', #52413, 1000.000000000000227 ) ;
#57610=AXIS2_PLACEMENT_3D ( 'NONE', #25278, #59484, #42940 ) ;
#57619=EDGE_LOOP ( 'NONE', ( #13464, #43204, #22734, #73393 ) ) ;
#57641=CARTESIAN_POINT ( 'NONE',  ( 8.700667342345820288, -98.11853780484867116, -2.500000000000000000 ) ) ;
#57674=DIRECTION ( 'NONE',  ( 1.000000000000000000, 0.000000000000000000, 0.000000000000000000 ) ) ;
#57679=SURFACE_STYLE_FILL_AREA ( #46387 ) ;
#57694=EDGE_LOOP ( 'NONE', ( #35311, #29693, #1837, #45871 ) ) ;
#57705=ORIENTED_EDGE ( 'NONE', *, *, #41581, .F. ) ;
#57724=EDGE_CURVE ( 'NONE', #19845, #45901, #8018, .T. ) ;
#57725=ORIENTED_EDGE ( 'NONE', *, *, #42983, .T. ) ;
#57738=VERTEX_POINT ( 'NONE', #63702 ) ;
#57756=CARTESIAN_POINT ( 'NONE',  ( 26.28306158492127764, -123.3838844133976522, 2.500000000000000000 ) ) ;
#57782=DIRECTION ( 'NONE',  ( 1.000000000000000000, 0.000000000000000000, 0.000000000000000000 ) ) ;
#57819=LINE ( 'NONE', #36350, #53759 ) ;
#57831=EDGE_LOOP ( 'NONE', ( #67544, #16459, #29738, #5846 ) ) ;
#57837=DIRECTION ( 'NONE',  ( -0.9730327541852497042, 0.2306669878475623159, 0.000000000000000000 ) ) ;
#57863=DIRECTION ( 'NONE',  ( 0.1850432970638667407, -0.9827303690289282967, 0.000000000000000000 ) ) ;
#57877=EDGE_CURVE ( 'NONE', #19049, #27761, #20770, .T. ) ;
#57958=EDGE_LOOP ( 'NONE', ( #38351, #54465, #25148, #1279 ) ) ;
#57977=CARTESIAN_POINT ( 'NONE',  ( -24.50849501662245444, -109.8101191361138831, 2.500000000000000000 ) ) ;
#57995=CARTESIAN_POINT ( 'NONE',  ( 0.000000000000000000, -120.0000000000000000, 5.500000000000000888 ) ) ;
#58018=DIRECTION ( 'NONE',  ( -0.000000000000000000, -0.000000000000000000, -1.000000000000000000 ) ) ;
#58030=CARTESIAN_POINT ( 'NONE',  ( 16.30584220631899228, -140.9432449716519784, 5.500000000000000000 ) ) ;
#58034=VECTOR ( 'NONE', #2717, 1000.000000000000000 ) ;
#58053=DIRECTION ( 'NONE',  ( -0.4279312458752977388, -0.9038112904824853189, 0.000000000000000000 ) ) ;
#58060=ORIENTED_EDGE ( 'NONE', *, *, #37591, .T. ) ;
#58064=VERTEX_POINT ( 'NONE', #56102 ) ;
#58066=ORIENTED_EDGE ( 'NONE', *, *, #37534, .T. ) ;
#58091=EDGE_CURVE ( 'NONE', #11947, #55143, #22633, .T. ) ;
#58111=CARTESIAN_POINT ( 'NONE',  ( -21.33958957442910886, -129.9559990355020034, -5.500000000000000000 ) ) ;
#58114=EDGE_LOOP ( 'NONE', ( #62115, #39537, #4181, #49627 ) ) ;
#58127=PLANE ( 'NONE',  #15406 ) ;
#58141=CARTESIAN_POINT ( 'NONE',  ( -16.06301359042743115, -102.7814171781257357, 5.500000000000000000 ) ) ;
#58146=ORIENTED_EDGE ( 'NONE', *, *, #43389, .T. ) ;
#58151=AXIS2_PLACEMENT_3D ( 'NONE', #39480, #57511, #16164 ) ;
#58155=CARTESIAN_POINT ( 'NONE',  ( -18.12185313557660038, -104.9634299478706794, 5.500000000000000000 ) ) ;
#58167=CARTESIAN_POINT ( 'NONE',  ( -26.29030328629083968, -123.6496510949466341, 5.500000000000000000 ) ) ;
#58203=CARTESIAN_POINT ( 'NONE',  ( -26.53422223201112828, -120.6595836127786043, 5.500000000000000000 ) ) ;
#58218=DIRECTION ( 'NONE',  ( -0.000000000000000000, -0.000000000000000000, -1.000000000000000000 ) ) ;
#58220=EDGE_CURVE ( 'NONE', #28951, #42454, #25854, .T. ) ;
#58236=ADVANCED_FACE ( 'NONE', ( #30008 ), #36028, .T. ) ;
#58251=CARTESIAN_POINT ( 'NONE',  ( 23.41451323550360186, -132.5004227906269989, 5.500000000000000000 ) ) ;
#58256=PLANE ( 'NONE',  #13739 ) ;
#58275=EDGE_LOOP ( 'NONE', ( #7659, #34694 ) ) ;
#58303=AXIS2_PLACEMENT_3D ( 'NONE', #20825, #15182, #48293 ) ;
#58304=CARTESIAN_POINT ( 'NONE',  ( 0.000000000000000000, -120.0000000000000000, -2.500000000000000000 ) ) ;
#58345=CARTESIAN_POINT ( 'NONE',  ( 2.117611129180199558, -93.54218975225703048, 5.500000000000000000 ) ) ;
#58348=VECTOR ( 'NONE', #29410, 1000.000000000000000 ) ;
#58357=CARTESIAN_POINT ( 'NONE',  ( -19.90058851926621131, -132.5883508287165853, 2.500000000000000000 ) ) ;
#58367=ORIENTED_EDGE ( 'NONE', *, *, #69511, .T. ) ;
#58371=DIRECTION ( 'NONE',  ( -0.2306669878475622604, -0.9730327541852497042, 0.000000000000000000 ) ) ;
#58372=CARTESIAN_POINT ( 'NONE',  ( 9.984461079971730157, -95.40710393340120277, 5.500000000000000000 ) ) ;
#58382=EDGE_CURVE ( 'NONE', #49489, #11010, #56297, .T. ) ;
#58389=CARTESIAN_POINT ( 'NONE',  ( 2.117611129180199558, -93.54218975225703048, 5.500000000000000000 ) ) ;
#58411=VECTOR ( 'NONE', #21779, 1000.000000000000114 ) ;
#58438=AXIS2_PLACEMENT_3D ( 'NONE', #12524, #47488, #35461 ) ;
#58465=EDGE_CURVE ( 'NONE', #34514, #9311, #68320, .T. ) ;
#58486=DIRECTION ( 'NONE',  ( -0.2306669878475648139, -0.9730327541852491491, 0.000000000000000000 ) ) ;
#58515=CARTESIAN_POINT ( 'NONE',  ( 14.59956846177685996, -138.4757300459248484, -5.500000000000000000 ) ) ;
#58519=CARTESIAN_POINT ( 'NONE',  ( 0.000000000000000000, -120.0000000000000000, -2.500000000000000000 ) ) ;
#58521=ORIENTED_EDGE ( 'NONE', *, *, #55945, .F. ) ;
#58529=CARTESIAN_POINT ( 'NONE',  ( 0.000000000000000000, -120.0000000000000000, 5.500000000000000000 ) ) ;
#58543=PLANE ( 'NONE',  #13663 ) ;
#58549=LINE ( 'NONE', #18692, #58761 ) ;
#58566=PLANE ( 'NONE',  #18639 ) ;
#58574=CARTESIAN_POINT ( 'NONE',  ( -14.87942725330654348, -141.9795960975983178, -5.500000000000000000 ) ) ;
#58581=CARTESIAN_POINT ( 'NONE',  ( -19.90058851926621131, -132.5883508287165853, 5.500000000000000000 ) ) ;
#58614=VECTOR ( 'NONE', #14736, 1000.000000000000000 ) ;
#58664=EDGE_CURVE ( 'NONE', #19127, #1038, #51315, .T. ) ;
#58671=VECTOR ( 'NONE', #28382, 1000.000000000000114 ) ;
#58676=DIRECTION ( 'NONE',  ( -0.9730327541852497042, 0.2306669878475622604, 0.000000000000000000 ) ) ;
#58695=ORIENTED_EDGE ( 'NONE', *, *, #50351, .F. ) ;
#58705=VERTEX_POINT ( 'NONE', #16753 ) ;
#58711=DIRECTION ( 'NONE',  ( -0.4796670183876294291, 0.8774505977381983346, 0.000000000000000000 ) ) ;
#58713=ORIENTED_EDGE ( 'NONE', *, *, #55919, .T. ) ;
#58718=ORIENTED_EDGE ( 'NONE', *, *, #14188, .T. ) ;
#58761=VECTOR ( 'NONE', #7047, 1000.000000000000000 ) ;
#58762=ORIENTED_EDGE ( 'NONE', *, *, #39675, .F. ) ;
#58777=FACE_OUTER_BOUND ( 'NONE', #72924, .T. ) ;
#58781=VECTOR ( 'NONE', #69562, 1000.000000000000114 ) ;
#58799=ORIENTED_EDGE ( 'NONE', *, *, #36083, .F. ) ;
#58811=ORIENTED_EDGE ( 'NONE', *, *, #10287, .F. ) ;
#58815=CARTESIAN_POINT ( 'NONE',  ( 23.41451323550360186, -132.5004227906269989, 5.500000000000000000 ) ) ;
#58831=LINE ( 'NONE', #7330, #6278 ) ;
#58863=VECTOR ( 'NONE', #72316, 1000.000000000000114 ) ;
#58894=AXIS2_PLACEMENT_3D ( 'NONE', #25078, #43130, #2568 ) ;
#58896=EDGE_CURVE ( 'NONE', #71554, #71724, #18950, .T. ) ;
#58898=LINE ( 'NONE', #13752, #30000 ) ;
#58905=DIRECTION ( 'NONE',  ( 0.2306669878475647861, 0.9730327541852491491, 0.000000000000000000 ) ) ;
#58954=VECTOR ( 'NONE', #50895, 1000.000000000000114 ) ;
#58967=FACE_OUTER_BOUND ( 'NONE', #72542, .T. ) ;
#58970=DIRECTION ( 'NONE',  ( -0.000000000000000000, -0.000000000000000000, 1.000000000000000000 ) ) ;
#58972=AXIS2_PLACEMENT_3D ( 'NONE', #12712, #18721, #36757 ) ;
#59013=EDGE_CURVE ( 'NONE', #14636, #51420, #53545, .T. ) ;
#59018=FACE_BOUND ( 'NONE', #8902, .T. ) ;
#59021=EDGE_CURVE ( 'NONE', #23903, #42454, #8049, .T. ) ;
#59050=CARTESIAN_POINT ( 'NONE',  ( -19.90058851926621131, -132.5883508287165853, -5.500000000000000000 ) ) ;
#59061=AXIS2_PLACEMENT_3D ( 'NONE', #42850, #36095, #7530 ) ;
#59085=FACE_BOUND ( 'NONE', #72744, .T. ) ;
#59128=CARTESIAN_POINT ( 'NONE',  ( 22.08297821871651934, -111.8242998470044540, 5.500000000000000000 ) ) ;
#59138=DIRECTION ( 'NONE',  ( 0.1850432970638682395, -0.9827303690289279636, 0.000000000000000000 ) ) ;
#59140=CARTESIAN_POINT ( 'NONE',  ( 21.85433023846371370, -135.0628101570779620, 5.500000000000000000 ) ) ;
#59169=EDGE_CURVE ( 'NONE', #55103, #34880, #49740, .T. ) ;
#59219=LINE ( 'NONE', #64870, #10135 ) ;
#59253=EDGE_LOOP ( 'NONE', ( #6302, #1826, #61106, #33532 ) ) ;
#59262=CARTESIAN_POINT ( 'NONE',  ( 16.30584220631899228, -140.9432449716519784, 5.500000000000000000 ) ) ;
#59265=VECTOR ( 'NONE', #57, 1000.000000000000114 ) ;
#59286=EDGE_LOOP ( 'NONE', ( #52584, #72580, #35990, #34595 ) ) ;
#59324=CARTESIAN_POINT ( 'NONE',  ( 20.85212586905262100, -130.9402397935870965, 5.500000000000000000 ) ) ;
#59367=DIRECTION ( 'NONE',  ( 0.2867529058022011967, -0.9580045777625459946, 0.000000000000000000 ) ) ;
#59383=PLANE ( 'NONE',  #21244 ) ;
#59421=DIRECTION ( 'NONE',  ( -0.4796670183876317051, 0.8774505977381971134, 0.000000000000000000 ) ) ;
#59423=CARTESIAN_POINT ( 'NONE',  ( 2.117611129180199558, -93.54218975225703048, -2.500000000000000444 ) ) ;
#59428=VECTOR ( 'NONE', #73658, 1000.000000000000114 ) ;
#59447=VECTOR ( 'NONE', #72411, 1000.000000000000000 ) ;
#59450=EDGE_LOOP ( 'NONE', ( #33763, #56640, #20365, #34185 ) ) ;
#59457=CARTESIAN_POINT ( 'NONE',  ( -22.53294031248082163, -134.0273518838794757, 5.500000000000000000 ) ) ;
#59463=VECTOR ( 'NONE', #49889, 1000.000000000000114 ) ;
#59484=DIRECTION ( 'NONE',  ( 0.08130631524009970801, -0.9966891607226786576, 0.000000000000000000 ) ) ;
#59498=VERTEX_POINT ( 'NONE', #13599 ) ;
#59513=VECTOR ( 'NONE', #44135, 1000.000000000000000 ) ;
#59528=ORIENTED_EDGE ( 'NONE', *, *, #59699, .F. ) ;
#59541=CARTESIAN_POINT ( 'NONE',  ( 16.84844760790522855, -103.5491698323862124, 5.500000000000000000 ) ) ;
#59545=VECTOR ( 'NONE', #68255, 1000.000000000000000 ) ;
#59552=VECTOR ( 'NONE', #25381, 1000.000000000000114 ) ;
#59585=CARTESIAN_POINT ( 'NONE',  ( 11.41210121379328335, -99.40233154247455616, -5.500000000000000000 ) ) ;
#59590=EDGE_CURVE ( 'NONE', #52067, #27833, #26717, .T. ) ;
#59603=CIRCLE ( 'NONE', #54808, 30.50000000000000000 ) ;
#59605=DIRECTION ( 'NONE',  ( 0.9580045777625458836, 0.2867529058022011412, -0.000000000000000000 ) ) ;
#59658=ORIENTED_EDGE ( 'NONE', *, *, #37848, .T. ) ;
#59699=EDGE_CURVE ( 'NONE', #6205, #3726, #33854, .T. ) ;
#59710=VECTOR ( 'NONE', #26494, 1000.000000000000227 ) ;
#59758=VERTEX_POINT ( 'NONE', #51141 ) ;
#59762=FACE_OUTER_BOUND ( 'NONE', #37182, .T. ) ;
#59764=ORIENTED_EDGE ( 'NONE', *, *, #15505, .T. ) ;
#59778=CARTESIAN_POINT ( 'NONE',  ( -26.41226275915097332, -122.1546173538626761, -2.500000000000000000 ) ) ;
#59782=FACE_OUTER_BOUND ( 'NONE', #19307, .T. ) ;
#59810=DIRECTION ( 'NONE',  ( 0.9435911131814402886, -0.3311129884571281101, 0.000000000000000000 ) ) ;
#59816=EDGE_CURVE ( 'NONE', #48167, #40486, #20913, .T. ) ;
#59821=EDGE_LOOP ( 'NONE', ( #14871, #20130, #50189, #46148 ) ) ;
#59822=FACE_BOUND ( 'NONE', #60787, .T. ) ;
#59825=EDGE_CURVE ( 'NONE', #23125, #6148, #47723, .T. ) ;
#59839=VECTOR ( 'NONE', #65271, 1000.000000000000114 ) ;
#59846=PLANE ( 'NONE',  #36481 ) ;
#59854=LINE ( 'NONE', #15078, #53952 ) ;
#59862=PLANE ( 'NONE',  #57610 ) ;
#59872=FACE_OUTER_BOUND ( 'NONE', #66205, .T. ) ;
#59883=LINE ( 'NONE', #30178, #26197 ) ;
#59884=LINE ( 'NONE', #43701, #23002 ) ;
#59904=LINE ( 'NONE', #31305, #11728 ) ;
#59944=VECTOR ( 'NONE', #53304, 1000.000000000000114 ) ;
#59973=EDGE_LOOP ( 'NONE', ( #17369, #46968, #57096, #43397 ) ) ;
#59979=CARTESIAN_POINT ( 'NONE',  ( -25.50183398199384754, -112.6408924756582053, 5.500000000000000000 ) ) ;
#60020=DIRECTION ( 'NONE',  ( -0.8541291221503265474, 0.5200609990133007177, 0.000000000000000000 ) ) ;
#60031=EDGE_CURVE ( 'NONE', #43453, #56886, #50594, .T. ) ;
#60034=DIRECTION ( 'NONE',  ( -0.000000000000000000, -0.000000000000000000, -1.000000000000000000 ) ) ;
#60061=EDGE_CURVE ( 'NONE', #24488, #38008, #51334, .T. ) ;
#60100=ADVANCED_FACE ( 'NONE', ( #29140 ), #265, .F. ) ;
#60109=DIRECTION ( 'NONE',  ( 0.9730327541852493711, -0.2306669878475637314, 0.000000000000000000 ) ) ;
#60116=EDGE_LOOP ( 'NONE', ( #72403, #36926, #69978, #44318 ) ) ;
#60124=DIRECTION ( 'NONE',  ( 0.9997280174009349762, -0.02332147558787674158, 0.000000000000000000 ) ) ;
#60129=DIRECTION ( 'NONE',  ( 0.2306669878475647861, 0.9730327541852491491, 0.000000000000000000 ) ) ;
#60200=ORIENTED_EDGE ( 'NONE', *, *, #3284, .F. ) ;
#60208=EDGE_LOOP ( 'NONE', ( #68239, #30951, #41726, #12920 ) ) ;
#60210=CARTESIAN_POINT ( 'NONE',  ( -18.12185313557659683, -104.9634299478706794, -2.500000000000000000 ) ) ;
#60221=CARTESIAN_POINT ( 'NONE',  ( -0.9515373497862389396, -96.47140937769621871, -2.500000000000000000 ) ) ;
#60250=CARTESIAN_POINT ( 'NONE',  ( -7.670864526094549163, -97.73662565058241114, -5.500000000000000000 ) ) ;
#60253=ORIENTED_EDGE ( 'NONE', *, *, #10538, .F. ) ;
#60258=CARTESIAN_POINT ( 'NONE',  ( 2.047646702416564768, -96.54137380445985173, 5.500000000000000000 ) ) ;
#60274=EDGE_CURVE ( 'NONE', #47167, #63004, #8065, .T. ) ;
#60279=ORIENTED_EDGE ( 'NONE', *, *, #59590, .T. ) ;
#60321=DIRECTION ( 'NONE',  ( -0.000000000000000000, -0.000000000000000000, -1.000000000000000000 ) ) ;
#60333=PLANE ( 'NONE',  #23060 ) ;
#60354=ADVANCED_FACE ( 'NONE', ( #25366 ), #55037, .F. ) ;
#60355=PLANE ( 'NONE',  #11289 ) ;
#60387=DIRECTION ( 'NONE',  ( -0.000000000000000000, -0.000000000000000000, -1.000000000000000000 ) ) ;
#60397=ORIENTED_EDGE ( 'NONE', *, *, #36314, .T. ) ;
#60415=CARTESIAN_POINT ( 'NONE',  ( -17.09243336300205129, -103.8724235629982502, 2.500000000000000000 ) ) ;
#60419=VERTEX_POINT ( 'NONE', #67433 ) ;
#60440=DIRECTION ( 'NONE',  ( -0.9730327541852491491, 0.2306669878475648139, 0.000000000000000000 ) ) ;
#60476=ORIENTED_EDGE ( 'NONE', *, *, #52280, .T. ) ;
#60483=ORIENTED_EDGE ( 'NONE', *, *, #46700, .T. ) ;
#60524=VECTOR ( 'NONE', #32864, 1000.000000000000000 ) ;
#60554=EDGE_CURVE ( 'NONE', #71157, #32752, #5778, .T. ) ;
#60574=FACE_OUTER_BOUND ( 'NONE', #59286, .T. ) ;
#60597=DIRECTION ( 'NONE',  ( 0.6862798483830533369, 0.7273375899149812085, 0.000000000000000000 ) ) ;
#60598=ADVANCED_FACE ( 'NONE', ( #62938 ), #29058, .F. ) ;
#60612=DIRECTION ( 'NONE',  ( -0.3853207896976533764, 0.9227826878668546895, 0.000000000000000000 ) ) ;
#60635=EDGE_CURVE ( 'NONE', #54914, #27087, #30162, .T. ) ;
#60638=EDGE_CURVE ( 'NONE', #8157, #40486, #6152, .T. ) ;
#60705=CIRCLE ( 'NONE', #7826, 32.50000000000000000 ) ;
#60713=FACE_OUTER_BOUND ( 'NONE', #57519, .T. ) ;
#60717=PLANE ( 'NONE',  #27111 ) ;
#60728=AXIS2_PLACEMENT_3D ( 'NONE', #23156, #7339, #41542 ) ;
#60736=VECTOR ( 'NONE', #65953, 1000.000000000000114 ) ;
#60743=VECTOR ( 'NONE', #53846, 1000.000000000000000 ) ;
#60749=DIRECTION ( 'NONE',  ( -0.5687579148473743684, 0.8225049752423791993, 0.000000000000000000 ) ) ;
#60756=EDGE_CURVE ( 'NONE', #63983, #25489, #64763, .T. ) ;
#60762=EDGE_CURVE ( 'NONE', #34299, #14636, #19621, .T. ) ;
#60772=LINE ( 'NONE', #54383, #31416 ) ;
#60785=LINE ( 'NONE', #72770, #8719 ) ;
#60787=EDGE_LOOP ( 'NONE', ( #32975, #21143, #5268, #2145 ) ) ;
#60789=VECTOR ( 'NONE', #62962, 1000.000000000000114 ) ;
#60796=ORIENTED_EDGE ( 'NONE', *, *, #30377, .T. ) ;
#60807=DIRECTION ( 'NONE',  ( 0.8541291221503261033, -0.5200609990133016058, 0.000000000000000000 ) ) ;
#60853=ORIENTED_EDGE ( 'NONE', *, *, #42274, .T. ) ;
#60927=AXIS2_PLACEMENT_3D ( 'NONE', #73256, #55607, #48847 ) ;
#60935=ORIENTED_EDGE ( 'NONE', *, *, #39683, .F. ) ;
#60937=ORIENTED_EDGE ( 'NONE', *, *, #51102, .F. ) ;
#60947=ORIENTED_EDGE ( 'NONE', *, *, #28423, .F. ) ;
#60963=CARTESIAN_POINT ( 'NONE',  ( 11.41210121379328335, -99.40233154247455616, -5.500000000000000000 ) ) ;
#60990=FACE_OUTER_BOUND ( 'NONE', #9861, .T. ) ;
#60992=FACE_OUTER_BOUND ( 'NONE', #1539, .T. ) ;
#60994=DIRECTION ( 'NONE',  ( -0.7950889364178796992, 0.6064928550163510845, 0.000000000000000000 ) ) ;
#61059=AXIS2_PLACEMENT_3D ( 'NONE', #50545, #4714, #50918 ) ;
#61074=EDGE_LOOP ( 'NONE', ( #67785, #9628, #1438, #401 ) ) ;
#61106=ORIENTED_EDGE ( 'NONE', *, *, #66380, .T. ) ;
#61107=VECTOR ( 'NONE', #17521, 1000.000000000000227 ) ;
#61150=VECTOR ( 'NONE', #17469, 1000.000000000000114 ) ;
#61156=LINE ( 'NONE', #2924, #49272 ) ;
#61173=VECTOR ( 'NONE', #19696, 1000.000000000000114 ) ;
#61189=LINE ( 'NONE', #15312, #59463 ) ;
#61202=VERTEX_POINT ( 'NONE', #23345 ) ;
#61220=DIRECTION ( 'NONE',  ( 0.8774505977381971134, 0.4796670183876317051, -0.000000000000000000 ) ) ;
#61225=VECTOR ( 'NONE', #73688, 1000.000000000000114 ) ;
#61233=ORIENTED_EDGE ( 'NONE', *, *, #69082, .T. ) ;
#61244=FACE_OUTER_BOUND ( 'NONE', #50202, .T. ) ;
#61263=AXIS2_PLACEMENT_3D ( 'NONE', #33220, #27200, #50135 ) ;
#61267=CARTESIAN_POINT ( 'NONE',  ( -18.12185313557660038, -104.9634299478706794, 2.500000000000000000 ) ) ;
#61277=EDGE_CURVE ( 'NONE', #4157, #9311, #24444, .T. ) ;
#61279=ADVANCED_FACE ( 'NONE', ( #18789 ), #53388, .F. ) ;
#61293=CARTESIAN_POINT ( 'NONE',  ( 0.000000000000000000, -120.0000000000000000, 2.500000000000000000 ) ) ;
#61360=CARTESIAN_POINT ( 'NONE',  ( 4.348517481000897078, -143.0941636721797465, 2.500000000000000000 ) ) ;
#61377=CARTESIAN_POINT ( 'NONE',  ( 0.7195005275814480017, -121.3161758966073052, -2.500000000000000000 ) ) ;
#61380=CARTESIAN_POINT ( 'NONE',  ( 0.000000000000000000, -89.50000000000000000, 2.500000000000000000 ) ) ;
#61384=CARTESIAN_POINT ( 'NONE',  ( -3.961125083139900749, -143.2122702051246677, -2.500000000000000000 ) ) ;
#61397=EDGE_CURVE ( 'NONE', #68902, #31369, #27776, .T. ) ;
#61398=DIRECTION ( 'NONE',  ( 0.6516173805718078471, -0.7585478161175706058, 0.000000000000000000 ) ) ;
#61402=LINE ( 'NONE', #4266, #56380 ) ;
#61412=ORIENTED_EDGE ( 'NONE', *, *, #16462, .F. ) ;
#61414=AXIS2_PLACEMENT_3D ( 'NONE', #10873, #33798, #63495 ) ;
#61437=CARTESIAN_POINT ( 'NONE',  ( 25.81725066941077529, -113.8380548628854854, 5.500000000000000000 ) ) ;
#61445=DIRECTION ( 'NONE',  ( -0.6516173805718079581, 0.7585478161175706058, 0.000000000000000000 ) ) ;
#61457=LINE ( 'NONE', #25391, #40588 ) ;
#61469=ORIENTED_EDGE ( 'NONE', *, *, #55536, .F. ) ;
#61535=CARTESIAN_POINT ( 'NONE',  ( -21.67772167707813935, -110.8034581014852762, 5.500000000000000000 ) ) ;
#61570=DIRECTION ( 'NONE',  ( -0.000000000000000000, -0.000000000000000000, -1.000000000000000000 ) ) ;
#61587=DIRECTION ( 'NONE',  ( 0.000000000000000000, 0.000000000000000000, 1.000000000000000000 ) ) ;
#61612=EDGE_CURVE ( 'NONE', #9787, #62521, #63130, .T. ) ;
#61628=VECTOR ( 'NONE', #3519, 1000.000000000000000 ) ;
#61631=DIRECTION ( 'NONE',  ( -0.000000000000000000, -0.000000000000000000, -1.000000000000000000 ) ) ;
#61637=CARTESIAN_POINT ( 'NONE',  ( -13.05994868825747446, -139.5943292883446532, 5.500000000000000000 ) ) ;
#61647=CARTESIAN_POINT ( 'NONE',  ( 1.459549131277868561, -120.3460004817713411, -2.500000000000000000 ) ) ;
#61659=DIRECTION ( 'NONE',  ( 1.000000000000000000, 0.000000000000000000, 0.000000000000000000 ) ) ;
#61675=PLANE ( 'NONE',  #17259 ) ;
#61684=CARTESIAN_POINT ( 'NONE',  ( 22.63442173698368620, -133.7816164738524378, 2.500000000000000000 ) ) ;
#61708=PLANE ( 'NONE',  #12183 ) ;
#61713=EDGE_CURVE ( 'NONE', #63983, #34836, #2579, .T. ) ;
#61717=ORIENTED_EDGE ( 'NONE', *, *, #18535, .T. ) ;
#61727=ORIENTED_EDGE ( 'NONE', *, *, #57877, .T. ) ;
#61733=ADVANCED_FACE ( 'NONE', ( #30353 ), #12695, .F. ) ;
#61768=PLANE ( 'NONE',  #9613 ) ;
#61769=ORIENTED_EDGE ( 'NONE', *, *, #60756, .F. ) ;
#61799=VERTEX_POINT ( 'NONE', #27688 ) ;
#61808=PLANE ( 'NONE',  #69613 ) ;
#61824=EDGE_LOOP ( 'NONE', ( #55832, #65640 ) ) ;
#61827=DIRECTION ( 'NONE',  ( -0.02332147558787674158, -0.9997280174009349762, 0.000000000000000000 ) ) ;
#61868=VERTEX_POINT ( 'NONE', #72427 ) ;
#61873=CARTESIAN_POINT ( 'NONE',  ( -15.44521549751111422, -137.7748507232956001, 5.500000000000000000 ) ) ;
#61875=CARTESIAN_POINT ( 'NONE',  ( 30.50000000000000000, -120.0000000000000000, 2.500000000000000000 ) ) ;
#61879=LINE ( 'NONE', #28385, #13788 ) ;
#61895=CARTESIAN_POINT ( 'NONE',  ( 8.700667342345820288, -98.11853780484867116, -5.500000000000000000 ) ) ;
#61947=CARTESIAN_POINT ( 'NONE',  ( -6.112675177960399608, -145.7853679859090903, -2.500000000000000000 ) ) ;
#61954=ADVANCED_FACE ( 'NONE', ( #16544 ), #32705, .F. ) ;
#61960=PLANE ( 'NONE',  #54962 ) ;
#61973=VECTOR ( 'NONE', #44897, 1000.000000000000227 ) ;
#61988=ORIENTED_EDGE ( 'NONE', *, *, #72724, .T. ) ;
#61989=COLOUR_RGB ( '', 0.09019608, 0.27058824, 0.51372549) ;
#62006=CARTESIAN_POINT ( 'NONE',  ( -10.43921258969510824, -98.89258801967538659, -5.500000000000000000 ) ) ;
#62033=CARTESIAN_POINT ( 'NONE',  ( -18.24502636017238899, -100.7225776329765665, 5.500000000000000000 ) ) ;
#62037=ORIENTED_EDGE ( 'NONE', *, *, #16061, .F. ) ;
#62064=ORIENTED_EDGE ( 'NONE', *, *, #59169, .T. ) ;
#62072=CARTESIAN_POINT ( 'NONE',  ( 0.000000000000000000, -89.50000000000000000, -2.500000000000000000 ) ) ;
#62093=DIRECTION ( 'NONE',  ( -0.08130631524010117905, 0.9966891607226784355, 0.000000000000000000 ) ) ;
#62095=DIRECTION ( 'NONE',  ( -0.6064928550163533050, -0.7950889364178781449, 0.000000000000000000 ) ) ;
#62102=LINE ( 'NONE', #22247, #4570 ) ;
#62111=PLANE ( 'NONE',  #23875 ) ;
#62115=ORIENTED_EDGE ( 'NONE', *, *, #55617, .F. ) ;
#62132=ORIENTED_EDGE ( 'NONE', *, *, #23360, .F. ) ;
#62141=EDGE_CURVE ( 'NONE', #65921, #17019, #780, .T. ) ;
#62156=CARTESIAN_POINT ( 'NONE',  ( -21.67772167707813935, -110.8034581014852762, -2.500000000000000000 ) ) ;
#62187=LINE ( 'NONE', #17067, #58954 ) ;
#62192=DIRECTION ( 'NONE',  ( 0.6516173805718058487, -0.7585478161175724932, 0.000000000000000000 ) ) ;
#62195=CARTESIAN_POINT ( 'NONE',  ( -7.670864526094549163, -97.73662565058241114, 2.500000000000000000 ) ) ;
#62222=LINE ( 'NONE', #10708, #12350 ) ;
#62224=AXIS2_PLACEMENT_3D ( 'NONE', #27968, #4698, #68206 ) ;
#62227=VECTOR ( 'NONE', #58018, 1000.000000000000000 ) ;
#62237=DIRECTION ( 'NONE',  ( -0.3853207896976523772, 0.9227826878668550226, 0.000000000000000000 ) ) ;
#62254=AXIS2_PLACEMENT_3D ( 'NONE', #10409, #8279, #56667 ) ;
#62258=CARTESIAN_POINT ( 'NONE',  ( 32.50000000000000000, -120.0000000000000000, 2.500000000000000000 ) ) ;
#62264=ORIENTED_EDGE ( 'NONE', *, *, #55322, .F. ) ;
#62268=FACE_OUTER_BOUND ( 'NONE', #17309, .T. ) ;
#62271=EDGE_LOOP ( 'NONE', ( #47067, #5874, #33652, #21511 ) ) ;
#62287=CARTESIAN_POINT ( 'NONE',  ( 48.80839716909466830, -10.37454508288725208, -5.500000000000000000 ) ) ;
#62296=LINE ( 'NONE', #21682, #22038 ) ;
#62309=EDGE_CURVE ( 'NONE', #36390, #46172, #14972, .T. ) ;
#62310=VECTOR ( 'NONE', #7935, 1000.000000000000227 ) ;
#62316=EDGE_CURVE ( 'NONE', #33390, #11562, #65012, .T. ) ;
#62341=CARTESIAN_POINT ( 'NONE',  ( 18.80329974962065265, -105.8248132807389084, 2.500000000000000000 ) ) ;
#62342=ADVANCED_FACE ( 'NONE', ( #70992 ), #19494, .F. ) ;
#62347=EDGE_LOOP ( 'NONE', ( #17340, #55301, #55780, #25906 ) ) ;
#62360=CARTESIAN_POINT ( 'NONE',  ( -0.9515373497862389396, -96.47140937769621871, -5.500000000000000000 ) ) ;
#62361=VECTOR ( 'NONE', #60612, 999.9999999999998863 ) ;
#62364=CARTESIAN_POINT ( 'NONE',  ( -22.17439115976385366, -112.2188447712574799, 2.500000000000000000 ) ) ;
#62373=VECTOR ( 'NONE', #65008, 1000.000000000000000 ) ;
#62390=FACE_OUTER_BOUND ( 'NONE', #40215, .T. ) ;
#62401=AXIS2_PLACEMENT_3D ( 'NONE', #41660, #58970, #64987 ) ;
#62410=ADVANCED_FACE ( 'NONE', ( #57065 ), #45040, .F. ) ;
#62412=ADVANCED_FACE ( 'NONE', ( #28103 ), #55938, .T. ) ;
#62465=VERTEX_POINT ( 'NONE', #62341 ) ;
#62482=DIRECTION ( 'NONE',  ( -0.000000000000000000, -0.000000000000000000, -1.000000000000000000 ) ) ;
#62485=DIRECTION ( 'NONE',  ( -0.9435911131814402886, 0.3311129884571281101, 0.000000000000000000 ) ) ;
#62488=ADVANCED_FACE ( 'NONE', ( #43930 ), #61960, .F. ) ;
#62493=PLANE ( 'NONE',  #37602 ) ;
#62519=ORIENTED_EDGE ( 'NONE', *, *, #45267, .F. ) ;
#62521=VERTEX_POINT ( 'NONE', #35590 ) ;
#62580=DIRECTION ( 'NONE',  ( 0.000000000000000000, 0.000000000000000000, 1.000000000000000000 ) ) ;
#62593=LINE ( 'NONE', #51660, #17059 ) ;
#62614=EDGE_LOOP ( 'NONE', ( #71546, #62624, #56172, #16102 ) ) ;
#62624=ORIENTED_EDGE ( 'NONE', *, *, #41926, .F. ) ;
#62676=AXIS2_PLACEMENT_3D ( 'NONE', #27873, #62485, #56079 ) ;
#62682=DIRECTION ( 'NONE',  ( 0.9435911131814398445, -0.3311129884571295534, 0.000000000000000000 ) ) ;
#62687=VECTOR ( 'NONE', #35515, 1000.000000000000114 ) ;
#62688=EDGE_CURVE ( 'NONE', #28347, #69250, #42724, .T. ) ;
#62691=CARTESIAN_POINT ( 'NONE',  ( -5.420674214417706693, -142.8662697233533265, 2.500000000000000000 ) ) ;
#62698=VECTOR ( 'NONE', #68359, 1000.000000000000000 ) ;
#62735=ORIENTED_EDGE ( 'NONE', *, *, #8857, .T. ) ;
#62751=ORIENTED_EDGE ( 'NONE', *, *, #12660, .T. ) ;
#62762=ORIENTED_EDGE ( 'NONE', *, *, #65801, .F. ) ;
#62795=CARTESIAN_POINT ( 'NONE',  ( 14.59956846177685996, -138.4757300459248484, 5.500000000000000000 ) ) ;
#62804=DIRECTION ( 'NONE',  ( 0.9038112904824853189, -0.4279312458752977388, 0.000000000000000000 ) ) ;
#62812=DIRECTION ( 'NONE',  ( -0.6516173805718067369, 0.7585478161175716050, 0.000000000000000000 ) ) ;
#62813=DIRECTION ( 'NONE',  ( 1.000000000000000000, 0.000000000000000000, 0.000000000000000000 ) ) ;
#62855=VECTOR ( 'NONE', #39450, 1000.000000000000114 ) ;
#62868=ADVANCED_FACE ( 'NONE', ( #21634 ), #73502, .F. ) ;
#62881=PRODUCT_DEFINITION_FORMATION_WITH_SPECIFIED_SOURCE ( 'ANY', '', #37366, .NOT_KNOWN. ) ;
#62909=EDGE_CURVE ( 'NONE', #7483, #27087, #17482, .T. ) ;
#62936=EDGE_CURVE ( 'NONE', #52621, #63423, #40795, .T. ) ;
#62938=FACE_OUTER_BOUND ( 'NONE', #9320, .T. ) ;
#62951=EDGE_CURVE ( 'NONE', #71724, #19049, #40046, .T. ) ;
#62956=VECTOR ( 'NONE', #37915, 1000.000000000000000 ) ;
#62962=DIRECTION ( 'NONE',  ( 0.8774505977381983346, 0.4796670183876293736, 0.000000000000000000 ) ) ;
#62992=DIRECTION ( 'NONE',  ( -0.000000000000000000, -0.000000000000000000, -1.000000000000000000 ) ) ;
#62993=EDGE_CURVE ( 'NONE', #34951, #73248, #47169, .T. ) ;
#63004=VERTEX_POINT ( 'NONE', #28757 ) ;
#63043=ORIENTED_EDGE ( 'NONE', *, *, #56744, .F. ) ;
#63045=VECTOR ( 'NONE', #40887, 1000.000000000000000 ) ;
#63087=ADVANCED_FACE ( 'NONE', ( #8791 ), #20444, .F. ) ;
#63090=ORIENTED_EDGE ( 'NONE', *, *, #37887, .T. ) ;
#63124=DIRECTION ( 'NONE',  ( 0.7950889364178796992, -0.6064928550163510845, 0.000000000000000000 ) ) ;
#63130=LINE ( 'NONE', #40920, #9231 ) ;
#63158=VERTEX_POINT ( 'NONE', #54292 ) ;
#63170=ORIENTED_EDGE ( 'NONE', *, *, #22990, .F. ) ;
#63256=ORIENTED_EDGE ( 'NONE', *, *, #47515, .F. ) ;
#63265=ORIENTED_EDGE ( 'NONE', *, *, #45267, .T. ) ;
#63283=VECTOR ( 'NONE', #26067, 1000.000000000000000 ) ;
#63290=CARTESIAN_POINT ( 'NONE',  ( -25.00516449930816876, -111.2255058058861010, 2.500000000000000000 ) ) ;
#63301=CARTESIAN_POINT ( 'NONE',  ( 9.984461079971730157, -95.40710393340120277, 5.500000000000000000 ) ) ;
#63309=ORIENTED_EDGE ( 'NONE', *, *, #36815, .F. ) ;
#63314=FACE_OUTER_BOUND ( 'NONE', #3526, .T. ) ;
#63327=ORIENTED_EDGE ( 'NONE', *, *, #36405, .T. ) ;
#63357=ORIENTED_EDGE ( 'NONE', *, *, #65863, .T. ) ;
#63409=AXIS2_PLACEMENT_3D ( 'NONE', #73589, #61587, #34120 ) ;
#63423=VERTEX_POINT ( 'NONE', #22691 ) ;
#63443=DIRECTION ( 'NONE',  ( 0.000000000000000000, 0.000000000000000000, 1.000000000000000000 ) ) ;
#63495=DIRECTION ( 'NONE',  ( 0.1276937514489679404, 0.9918136447140103451, 0.000000000000000000 ) ) ;
#63499=FACE_OUTER_BOUND ( 'NONE', #14541, .T. ) ;
#63506=ADVANCED_FACE ( 'NONE', ( #2752 ), #42564, .F. ) ;
#63516=ADVANCED_FACE ( 'NONE', ( #26001 ), #8350, .F. ) ;
#63541=AXIS2_PLACEMENT_3D ( 'NONE', #40591, #34205, #68804 ) ;
#63569=ORIENTED_EDGE ( 'NONE', *, *, #40770, .F. ) ;
#63601=LINE ( 'NONE', #28991, #73038 ) ;
#63604=AXIS2_PLACEMENT_3D ( 'NONE', #57062, #5198, #64093 ) ;
#63608=FACE_OUTER_BOUND ( 'NONE', #3718, .T. ) ;
#63611=DIRECTION ( 'NONE',  ( -0.7950889364178798102, 0.6064928550163511956, 0.000000000000000000 ) ) ;
#63619=DIRECTION ( 'NONE',  ( 0.000000000000000000, 0.000000000000000000, 1.000000000000000000 ) ) ;
#63650=PLANE ( 'NONE',  #2868 ) ;
#63654=PLANE ( 'NONE',  #26296 ) ;
#63676=EDGE_CURVE ( 'NONE', #71724, #68795, #66604, .T. ) ;
#63686=VECTOR ( 'NONE', #64590, 1000.000000000000114 ) ;
#63699=ORIENTED_EDGE ( 'NONE', *, *, #40826, .T. ) ;
#63702=CARTESIAN_POINT ( 'NONE',  ( 16.84844760790522855, -103.5491698323862124, -5.500000000000000000 ) ) ;
#63710=CARTESIAN_POINT ( 'NONE',  ( 3.429551818649054340, -146.3199197248623875, -5.500000000000000000 ) ) ;
#63764=ORIENTED_EDGE ( 'NONE', *, *, #53986, .F. ) ;
#63766=EDGE_CURVE ( 'NONE', #19845, #56042, #811, .T. ) ;
#63774=CARTESIAN_POINT ( 'NONE',  ( -7.572224309238338336, -145.4393675041377492, 5.500000000000000000 ) ) ;
#63831=ORIENTED_EDGE ( 'NONE', *, *, #53495, .T. ) ;
#63848=ORIENTED_EDGE ( 'NONE', *, *, #52015, .F. ) ;
#63852=DIRECTION ( 'NONE',  ( 0.4279312458753000703, 0.9038112904824842087, 0.000000000000000000 ) ) ;
#63880=CARTESIAN_POINT ( 'NONE',  ( 0.4301293587033142574, -121.4370068666438556, 2.500000000000000000 ) ) ;
#63885=CARTESIAN_POINT ( 'NONE',  ( 5.822613034544236399, -142.8165987265839760, -5.500000000000000000 ) ) ;
#63891=VECTOR ( 'NONE', #16510, 1000.000000000000000 ) ;
#63904=FACE_OUTER_BOUND ( 'NONE', #34015, .T. ) ;
#63907=ORIENTED_EDGE ( 'NONE', *, *, #48196, .F. ) ;
#63916=VERTEX_POINT ( 'NONE', #19528 ) ;
#63972=CARTESIAN_POINT ( 'NONE',  ( -22.67106064244953245, -113.6342314410295842, 5.500000000000000000 ) ) ;
#63983=VERTEX_POINT ( 'NONE', #1553 ) ;
#63985=CARTESIAN_POINT ( 'NONE',  ( 11.41210121379327980, -99.40233154247455616, -2.500000000000000000 ) ) ;
#63994=EDGE_LOOP ( 'NONE', ( #60853, #67007, #35899, #6560 ) ) ;
#63997=ORIENTED_EDGE ( 'NONE', *, *, #48054, .F. ) ;
#64018=LINE ( 'NONE', #1275, #44343 ) ;
#64043=CARTESIAN_POINT ( 'NONE',  ( -21.67772167707813935, -110.8034581014852762, 5.500000000000000000 ) ) ;
#64049=PLANE ( 'NONE',  #58438 ) ;
#64057=LINE ( 'NONE', #12531, #53319 ) ;
#64060=VECTOR ( 'NONE', #54001, 1000.000000000000000 ) ;
#64093=DIRECTION ( 'NONE',  ( 0.000000000000000000, 0.000000000000000000, 1.000000000000000000 ) ) ;
#64095=VERTEX_POINT ( 'NONE', #47602 ) ;
#64126=ADVANCED_FACE ( 'NONE', ( #20131 ), #31042, .F. ) ;
#64140=LINE ( 'NONE', #29526, #30813 ) ;
#64142=CARTESIAN_POINT ( 'NONE',  ( -23.30023580412278505, -123.4057321492263384, -5.500000000000000000 ) ) ;
#64147=AXIS2_PLACEMENT_3D ( 'NONE', #61535, #3300, #25463 ) ;
#64159=VECTOR ( 'NONE', #4090, 1000.000000000000114 ) ;
#64173=LINE ( 'NONE', #69793, #57257 ) ;
#64174=VECTOR ( 'NONE', #25866, 1000.000000000000114 ) ;
#64209=EDGE_CURVE ( 'NONE', #23556, #64095, #58898, .T. ) ;
#64236=LINE ( 'NONE', #28521, #6305 ) ;
#64241=CARTESIAN_POINT ( 'NONE',  ( 26.47460221209471598, -121.8961639463267090, 5.500000000000000000 ) ) ;
#64243=PLANE ( 'NONE',  #67152 ) ;
#64252=ADVANCED_FACE ( 'NONE', ( #45964 ), #39200, .F. ) ;
#64263=AXIS2_PLACEMENT_3D ( 'NONE', #46875, #24310, #6287 ) ;
#64269=ORIENTED_EDGE ( 'NONE', *, *, #44074, .T. ) ;
#64270=AXIS2_PLACEMENT_3D ( 'NONE', #48058, #41670, #47322 ) ;
#64273=CARTESIAN_POINT ( 'NONE',  ( 12.69589495141918611, -96.69089767102708777, 5.500000000000000000 ) ) ;
#64331=ADVANCED_FACE ( 'NONE', ( #22280 ), #61768, .F. ) ;
#64337=EDGE_LOOP ( 'NONE', ( #22219, #20462, #34664, #46976 ) ) ;
#64355=VERTEX_POINT ( 'NONE', #10246 ) ;
#64365=EDGE_CURVE ( 'NONE', #23903, #40406, #5006, .T. ) ;
#64371=VECTOR ( 'NONE', #71117, 1000.000000000000227 ) ;
#64422=( LENGTH_UNIT ( ) NAMED_UNIT ( * ) SI_UNIT ( .MILLI., .METRE. ) );
#64431=CARTESIAN_POINT ( 'NONE',  ( -1.192633404626841198, -119.0902607174754451, 2.500000000000000000 ) ) ;
#64479=DIRECTION ( 'NONE',  ( 0.9580045777625452175, 0.2867529058022035837, -0.000000000000000000 ) ) ;
#64480=VECTOR ( 'NONE', #68057, 1000.000000000000000 ) ;
#64505=DIRECTION ( 'NONE',  ( -0.8225049752423776450, -0.5687579148473765889, 0.000000000000000000 ) ) ;
#64577=DIRECTION ( 'NONE',  ( -0.6064928550163533050, -0.7950889364178781449, 0.000000000000000000 ) ) ;
#64590=DIRECTION ( 'NONE',  ( 0.6064928550163531940, 0.7950889364178782559, 0.000000000000000000 ) ) ;
#64599=FACE_OUTER_BOUND ( 'NONE', #68040, .T. ) ;
#64602=CIRCLE ( 'NONE', #26157, 30.50000000000000000 ) ;
#64633=DIRECTION ( 'NONE',  ( 0.9038112904824853189, -0.4279312458752977388, 0.000000000000000000 ) ) ;
#64669=DIRECTION ( 'NONE',  ( -0.9827303690289279636, -0.1850432970638682117, 0.000000000000000000 ) ) ;
#64675=DIRECTION ( 'NONE',  ( -0.000000000000000000, -0.000000000000000000, -1.000000000000000000 ) ) ;
#64704=VECTOR ( 'NONE', #50885, 1000.000000000000000 ) ;
#64722=FACE_BOUND ( 'NONE', #7196, .T. ) ;
#64727=CARTESIAN_POINT ( 'NONE',  ( 23.11608002360578240, -124.4885236261218182, 5.500000000000000000 ) ) ;
#64729=VERTEX_POINT ( 'NONE', #57641 ) ;
#64738=VECTOR ( 'NONE', #62992, 1000.000000000000000 ) ;
#64763=LINE ( 'NONE', #54584, #64371 ) ;
#64773=VECTOR ( 'NONE', #57344, 999.9999999999998863 ) ;
#64781=LINE ( 'NONE', #47842, #74231 ) ;
#64794=( NAMED_UNIT ( * ) SI_UNIT ( $, .STERADIAN. ) SOLID_ANGLE_UNIT ( ) );
#64810=CARTESIAN_POINT ( 'NONE',  ( -26.53422223201112828, -120.6595836127786043, 2.500000000000000000 ) ) ;
#64830=CARTESIAN_POINT ( 'NONE',  ( 18.80329974962065265, -105.8248132807389084, 5.500000000000000000 ) ) ;
#64834=ADVANCED_FACE ( 'NONE', ( #36166 ), #63654, .T. ) ;
#64847=EDGE_CURVE ( 'NONE', #33390, #46803, #64018, .T. ) ;
#64853=CARTESIAN_POINT ( 'NONE',  ( 22.94323693612312809, -114.6983135802921083, -5.500000000000000000 ) ) ;
#64870=CARTESIAN_POINT ( 'NONE',  ( 11.41210121379328335, -99.40233154247455616, 5.500000000000000000 ) ) ;
#64872=ADVANCED_FACE ( 'NONE', ( #55311 ), #14348, .F. ) ;
#64883=LINE ( 'NONE', #17895, #20512 ) ;
#64889=EDGE_CURVE ( 'NONE', #56961, #70524, #59854, .T. ) ;
#64930=DIRECTION ( 'NONE',  ( 1.000000000000000000, 0.000000000000000000, 0.000000000000000000 ) ) ;
#64962=VERTEX_POINT ( 'NONE', #36907 ) ;
#64986=AXIS2_PLACEMENT_3D ( 'NONE', #40074, #29509, #5876 ) ;
#64987=DIRECTION ( 'NONE',  ( 1.000000000000000000, 0.000000000000000000, 0.000000000000000000 ) ) ;
#64995=LINE ( 'NONE', #4347, #23642 ) ;
#65008=DIRECTION ( 'NONE',  ( -0.000000000000000000, -0.000000000000000000, -1.000000000000000000 ) ) ;
#65012=LINE ( 'NONE', #13847, #23729 ) ;
#65028=ORIENTED_EDGE ( 'NONE', *, *, #55322, .T. ) ;
#65034=DIRECTION ( 'NONE',  ( 0.000000000000000000, -0.000000000000000000, 1.000000000000000000 ) ) ;
#65088=ORIENTED_EDGE ( 'NONE', *, *, #49505, .T. ) ;
#65127=DIRECTION ( 'NONE',  ( 0.1276937514489679404, 0.9918136447140103451, -0.000000000000000000 ) ) ;
#65147=CARTESIAN_POINT ( 'NONE',  ( 21.85433023846371370, -135.0628101570779620, 5.500000000000000000 ) ) ;
#65178=EDGE_CURVE ( 'NONE', #14992, #70524, #69915, .T. ) ;
#65201=EDGE_CURVE ( 'NONE', #26020, #33066, #29319, .T. ) ;
#65244=ORIENTED_EDGE ( 'NONE', *, *, #40419, .F. ) ;
#65253=CARTESIAN_POINT ( 'NONE',  ( -0.4301293587032979371, -118.5629931333561871, 2.500000000000000000 ) ) ;
#65268=ORIENTED_EDGE ( 'NONE', *, *, #33415, .T. ) ;
#65271=DIRECTION ( 'NONE',  ( -0.5200609990132993854, -0.8541291221503275466, 0.000000000000000000 ) ) ;
#65285=VECTOR ( 'NONE', #48172, 1000.000000000000000 ) ;
#65294=VERTEX_POINT ( 'NONE', #24081 ) ;
#65326=CARTESIAN_POINT ( 'NONE',  ( 16.30584220631899228, -140.9432449716519784, -5.500000000000000000 ) ) ;
#65332=CARTESIAN_POINT ( 'NONE',  ( 0.000000000000000000, -120.0000000000000000, -2.500000000000000000 ) ) ;
#65354=EDGE_CURVE ( 'NONE', #55116, #60419, #36813, .T. ) ;
#65379=ADVANCED_FACE ( 'NONE', ( #59762 ), #30793, .F. ) ;
#65402=LINE ( 'NONE', #48463, #67269 ) ;
#65404=FACE_BOUND ( 'NONE', #57831, .T. ) ;
#65427=CARTESIAN_POINT ( 'NONE',  ( -23.54415474984308787, -120.4156646670583086, 2.500000000000000000 ) ) ;
#65448=CARTESIAN_POINT ( 'NONE',  ( 24.94940289813197509, -237.3777120880564553, 5.500000000000000000 ) ) ;
#65464=ORIENTED_EDGE ( 'NONE', *, *, #49036, .F. ) ;
#65468=FACE_BOUND ( 'NONE', #35805, .T. ) ;
#65493=EDGE_LOOP ( 'NONE', ( #49090, #21958, #29118, #63327 ) ) ;
#65500=ORIENTED_EDGE ( 'NONE', *, *, #74108, .T. ) ;
#65510=LINE ( 'NONE', #2759, #7387 ) ;
#65511=CARTESIAN_POINT ( 'NONE',  ( -26.41226275915097332, -122.1546173538626761, 2.500000000000000000 ) ) ;
#65520=CARTESIAN_POINT ( 'NONE',  ( -3.961125083139900749, -143.2122702051246677, 2.500000000000000000 ) ) ;
#65550=DIRECTION ( 'NONE',  ( -0.000000000000000000, -0.000000000000000000, -1.000000000000000000 ) ) ;
#65554=ORIENTED_EDGE ( 'NONE', *, *, #12645, .F. ) ;
#65579=DIRECTION ( 'NONE',  ( 0.7950889364178796992, -0.6064928550163510845, 0.000000000000000000 ) ) ;
#65580=STYLED_ITEM ( 'NONE', ( #24129 ), #37782 ) ;
#65595=DIRECTION ( 'NONE',  ( 0.000000000000000000, 0.000000000000000000, 1.000000000000000000 ) ) ;
#65640=ORIENTED_EDGE ( 'NONE', *, *, #4042, .T. ) ;
#65679=DIRECTION ( 'NONE',  ( -0.9580045777625456616, -0.2867529058022021404, 0.000000000000000000 ) ) ;
#65687=DIRECTION ( 'NONE',  ( -0.1276937514489679404, -0.9918136447140103451, 0.000000000000000000 ) ) ;
#65694=DIRECTION ( 'NONE',  ( -0.7950889364178781449, 0.6064928550163533050, 0.000000000000000000 ) ) ;
#65712=DIRECTION ( 'NONE',  ( -0.6862798483830534479, -0.7273375899149810975, 0.000000000000000000 ) ) ;
#65717=LINE ( 'NONE', #25486, #45593 ) ;
#65729=ORIENTED_EDGE ( 'NONE', *, *, #61612, .F. ) ;
#65744=EDGE_LOOP ( 'NONE', ( #8390, #7018, #57174, #19726 ) ) ;
#65779=CARTESIAN_POINT ( 'NONE',  ( -23.30023580412278505, -123.4057321492263384, 5.500000000000000000 ) ) ;
#65801=EDGE_CURVE ( 'NONE', #45219, #8157, #8158, .T. ) ;
#65829=DIRECTION ( 'NONE',  ( 1.000000000000000000, 0.000000000000000000, -0.000000000000000000 ) ) ;
#65840=CARTESIAN_POINT ( 'NONE',  ( 24.95699195200417364, -110.9640411295978595, -2.500000000000000000 ) ) ;
#65863=EDGE_CURVE ( 'NONE', #22041, #55469, #55137, .T. ) ;
#65867=ORIENTED_EDGE ( 'NONE', *, *, #24199, .F. ) ;
#65880=EDGE_CURVE ( 'NONE', #20073, #1781, #16682, .T. ) ;
#65892=DIRECTION ( 'NONE',  ( -0.000000000000000000, -0.000000000000000000, -1.000000000000000000 ) ) ;
#65902=VECTOR ( 'NONE', #60129, 1000.000000000000114 ) ;
#65909=AXIS2_PLACEMENT_3D ( 'NONE', #51932, #23375, #35020 ) ;
#65921=VERTEX_POINT ( 'NONE', #10661 ) ;
#65930=DIRECTION ( 'NONE',  ( -0.000000000000000000, -0.000000000000000000, -1.000000000000000000 ) ) ;
#65953=DIRECTION ( 'NONE',  ( 0.9997280174009349762, -0.02332147558787674158, 0.000000000000000000 ) ) ;
#66002=CARTESIAN_POINT ( 'NONE',  ( 12.13205353604972991, -140.1820037904669789, 5.500000000000000000 ) ) ;
#66022=DIRECTION ( 'NONE',  ( -0.000000000000000000, -0.000000000000000000, -1.000000000000000000 ) ) ;
#66043=DIRECTION ( 'NONE',  ( -1.000000000000000000, 0.000000000000000000, 0.000000000000000000 ) ) ;
#66049=ORIENTED_EDGE ( 'NONE', *, *, #54257, .F. ) ;
#66110=EDGE_CURVE ( 'NONE', #46803, #25695, #30900, .T. ) ;
#66112=EDGE_CURVE ( 'NONE', #26348, #17504, #40725, .T. ) ;
#66117=CARTESIAN_POINT ( 'NONE',  ( 22.08297821871651934, -111.8242998470044540, 5.500000000000000000 ) ) ;
#66126=CARTESIAN_POINT ( 'NONE',  ( 22.08297821871651934, -111.8242998470044540, -5.500000000000000000 ) ) ;
#66127=ORIENTED_EDGE ( 'NONE', *, *, #59699, .T. ) ;
#66128=FACE_OUTER_BOUND ( 'NONE', #64337, .T. ) ;
#66133=CARTESIAN_POINT ( 'NONE',  ( -10.21100092698785033, -95.54625877152835756, 2.500000000000000000 ) ) ;
#66154=LINE ( 'NONE', #67254, #69584 ) ;
#66162=PLANE ( 'NONE',  #19429 ) ;
#66169=DIRECTION ( 'NONE',  ( 0.9227826878668540234, 0.3853207896976547087, 0.000000000000000000 ) ) ;
#66205=EDGE_LOOP ( 'NONE', ( #48616, #3051, #44008, #41640 ) ) ;
#66209=FACE_BOUND ( 'NONE', #51527, .T. ) ;
#66224=EDGE_CURVE ( 'NONE', #68284, #9787, #55698, .T. ) ;
#66236=CARTESIAN_POINT ( 'NONE',  ( 2.117611129180199558, -93.54218975225703048, 5.500000000000000000 ) ) ;
#66256=ORIENTED_EDGE ( 'NONE', *, *, #14084, .T. ) ;
#66272=CARTESIAN_POINT ( 'NONE',  ( 20.07203437053270179, -132.2214334768125354, -2.500000000000000000 ) ) ;
#66282=CARTESIAN_POINT ( 'NONE',  ( -26.29030328629083968, -123.6496510949466341, 5.500000000000000000 ) ) ;
#66335=UNCERTAINTY_MEASURE_WITH_UNIT (LENGTH_MEASURE( 1.000000000000000082E-05 ), #47497, 'distance_accuracy_value', 'NONE');
#66380=EDGE_CURVE ( 'NONE', #24434, #34836, #32747, .T. ) ;
#66381=ADVANCED_FACE ( 'NONE', ( #59872 ), #51541, .F. ) ;
#66428=PLANE ( 'NONE',  #58894 ) ;
#66438=ORIENTED_EDGE ( 'NONE', *, *, #54477, .T. ) ;
#66451=LINE ( 'NONE', #13813, #6014 ) ;
#66458=VECTOR ( 'NONE', #67210, 1000.000000000000114 ) ;
#66463=AXIS2_PLACEMENT_3D ( 'NONE', #57158, #10528, #62813 ) ;
#66497=CARTESIAN_POINT ( 'NONE',  ( 20.85212586905262100, -130.9402397935870965, 5.500000000000000000 ) ) ;
#66550=DIRECTION ( 'NONE',  ( -0.000000000000000000, -0.000000000000000000, -1.000000000000000000 ) ) ;
#66559=ORIENTED_EDGE ( 'NONE', *, *, #66798, .F. ) ;
#66591=ORIENTED_EDGE ( 'NONE', *, *, #28496, .T. ) ;
#66604=LINE ( 'NONE', #15084, #2360 ) ;
#66616=CARTESIAN_POINT ( 'NONE',  ( -14.87942725330654348, -141.9795960975983178, -5.500000000000000000 ) ) ;
#66619=EDGE_CURVE ( 'NONE', #28408, #54047, #69930, .T. ) ;
#66631=CARTESIAN_POINT ( 'NONE',  ( 1.459549131277868561, -120.3460004817713411, 2.500000000000000000 ) ) ;
#66647=AXIS2_PLACEMENT_3D ( 'NONE', #63774, #40091, #5892 ) ;
#66660=CARTESIAN_POINT ( 'NONE',  ( -13.05994868825747446, -139.5943292883446532, 5.500000000000000000 ) ) ;
#66663=ORIENTED_EDGE ( 'NONE', *, *, #25650, .T. ) ;
#66666=ORIENTED_EDGE ( 'NONE', *, *, #45798, .F. ) ;
#66669=AXIS2_PLACEMENT_3D ( 'NONE', #3887, #38453, #25037 ) ;
#66751=ORIENTED_EDGE ( 'NONE', *, *, #37964, .F. ) ;
#66753=DIRECTION ( 'NONE',  ( 0.1850432970638656582, -0.9827303690289285187, 0.000000000000000000 ) ) ;
#66754=CARTESIAN_POINT ( 'NONE',  ( -26.53422223201112828, -120.6595836127786043, -2.500000000000000444 ) ) ;
#66760=ORIENTED_EDGE ( 'NONE', *, *, #11879, .T. ) ;
#66771=EDGE_LOOP ( 'NONE', ( #65554, #12274, #72640, #51026 ) ) ;
#66778=LINE ( 'NONE', #19794, #14197 ) ;
#66798=EDGE_CURVE ( 'NONE', #7707, #15838, #13889, .T. ) ;
#66810=CARTESIAN_POINT ( 'NONE',  ( -4.653126046682595884, -146.1313684676804314, 5.500000000000000000 ) ) ;
#66825=ADVANCED_FACE ( 'NONE', ( #31926 ), #54866, .F. ) ;
#66835=ORIENTED_EDGE ( 'NONE', *, *, #3191, .T. ) ;
#66962=ADVANCED_FACE ( 'NONE', ( #56365 ), #10865, .F. ) ;
#66989=DIRECTION ( 'NONE',  ( 1.000000000000000000, 0.000000000000000000, -0.000000000000000000 ) ) ;
#66998=DIRECTION ( 'NONE',  ( 0.8774505977381978905, 0.4796670183876304283, -0.000000000000000000 ) ) ;
#67005=VECTOR ( 'NONE', #48504, 1000.000000000000114 ) ;
#67007=ORIENTED_EDGE ( 'NONE', *, *, #41012, .T. ) ;
#67008=VECTOR ( 'NONE', #45489, 1000.000000000000000 ) ;
#67014=DIRECTION ( 'NONE',  ( -0.5200609990133016058, -0.8541291221503261033, 0.000000000000000000 ) ) ;
#67058=CARTESIAN_POINT ( 'NONE',  ( 2.047646702416564768, -96.54137380445985173, 5.500000000000000000 ) ) ;
#67065=ORIENTED_EDGE ( 'NONE', *, *, #68957, .F. ) ;
#67069=ADVANCED_FACE ( 'NONE', ( #35274 ), #58566, .F. ) ;
#67081=PLANE ( 'NONE',  #9137 ) ;
#67109=EDGE_CURVE ( 'NONE', #1173, #30034, #29608, .T. ) ;
#67113=VERTEX_POINT ( 'NONE', #41642 ) ;
#67125=ORIENTED_EDGE ( 'NONE', *, *, #9253, .T. ) ;
#67142=LINE ( 'NONE', #49840, #6221 ) ;
#67152=AXIS2_PLACEMENT_3D ( 'NONE', #36385, #25119, #42782 ) ;
#67182=VECTOR ( 'NONE', #41515, 1000.000000000000000 ) ;
#67195=ORIENTED_EDGE ( 'NONE', *, *, #24630, .T. ) ;
#67199=PLANE ( 'NONE',  #43183 ) ;
#67210=DIRECTION ( 'NONE',  ( 0.6064928550163524168, 0.7950889364178788110, -0.000000000000000000 ) ) ;
#67216=ORIENTED_EDGE ( 'NONE', *, *, #29282, .T. ) ;
#67217=LINE ( 'NONE', #64830, #52749 ) ;
#67244=ORIENTED_EDGE ( 'NONE', *, *, #13418, .F. ) ;
#67245=DIRECTION ( 'NONE',  ( -0.6516173805718079581, 0.7585478161175704948, 0.000000000000000000 ) ) ;
#67254=CARTESIAN_POINT ( 'NONE',  ( 1.499592026101426168, -120.0349822133818094, 2.500000000000000000 ) ) ;
#67269=VECTOR ( 'NONE', #13866, 999.9999999999998863 ) ;
#67272=CARTESIAN_POINT ( 'NONE',  ( 11.41210121379328335, -99.40233154247455616, 5.500000000000000000 ) ) ;
#67274=CARTESIAN_POINT ( 'NONE',  ( 19.29194287201271507, -133.5026271600380880, -2.500000000000000000 ) ) ;
#67280=LINE ( 'NONE', #15774, #23325 ) ;
#67291=EDGE_CURVE ( 'NONE', #1038, #56786, #29422, .T. ) ;
#67300=ORIENTED_EDGE ( 'NONE', *, *, #9193, .F. ) ;
#67312=ORIENTED_EDGE ( 'NONE', *, *, #15730, .F. ) ;
#67320=ORIENTED_EDGE ( 'NONE', *, *, #16762, .T. ) ;
#67326=ADVANCED_FACE ( 'NONE', ( #32201 ), #55894, .F. ) ;
#67332=CARTESIAN_POINT ( 'NONE',  ( -26.29030328629083968, -123.6496510949466341, 5.500000000000000000 ) ) ;
#67347=CARTESIAN_POINT ( 'NONE',  ( -23.97194136764370498, -131.3950000906648938, 5.500000000000000000 ) ) ;
#67385=ORIENTED_EDGE ( 'NONE', *, *, #65863, .F. ) ;
#67390=LINE ( 'NONE', #72639, #13838 ) ;
#67394=ORIENTED_EDGE ( 'NONE', *, *, #73766, .F. ) ;
#67405=LINE ( 'NONE', #50484, #44101 ) ;
#67407=ORIENTED_EDGE ( 'NONE', *, *, #33676, .T. ) ;
#67433=CARTESIAN_POINT ( 'NONE',  ( -23.97194136764370498, -131.3950000906648938, -2.500000000000000444 ) ) ;
#67463=ADVANCED_FACE ( 'NONE', ( #10024 ), #26937, .F. ) ;
#67464=VECTOR ( 'NONE', #4427, 1000.000000000000114 ) ;
#67470=EDGE_LOOP ( 'NONE', ( #42027, #72842, #14169, #70717 ) ) ;
#67510=LINE ( 'NONE', #73880, #28230 ) ;
#67511=DIRECTION ( 'NONE',  ( 0.3853207896976523772, -0.9227826878668550226, 0.000000000000000000 ) ) ;
#67520=ORIENTED_EDGE ( 'NONE', *, *, #74108, .F. ) ;
#67522=LINE ( 'NONE', #11485, #26217 ) ;
#67544=ORIENTED_EDGE ( 'NONE', *, *, #38968, .F. ) ;
#67584=FACE_OUTER_BOUND ( 'NONE', #10536, .T. ) ;
#67605=ORIENTED_EDGE ( 'NONE', *, *, #33731, .F. ) ;
#67611=DIRECTION ( 'NONE',  ( 0.7950889364178798102, -0.6064928550163511956, 0.000000000000000000 ) ) ;
#67659=DIRECTION ( 'NONE',  ( -0.4796670183876294291, 0.8774505977381983346, 0.000000000000000000 ) ) ;
#67674=AXIS2_PLACEMENT_3D ( 'NONE', #25262, #48185, #31257 ) ;
#67704=ORIENTED_EDGE ( 'NONE', *, *, #60031, .T. ) ;
#67737=ORIENTED_EDGE ( 'NONE', *, *, #18379, .F. ) ;
#67774=CARTESIAN_POINT ( 'NONE',  ( 8.700667342345820288, -98.11853780484867116, 5.500000000000000000 ) ) ;
#67785=ORIENTED_EDGE ( 'NONE', *, *, #29537, .F. ) ;
#67830=FACE_OUTER_BOUND ( 'NONE', #56797, .T. ) ;
#67838=ADVANCED_FACE ( 'NONE', ( #14086 ), #8467, .F. ) ;
#67891=ADVANCED_FACE ( 'NONE', ( #67830, #72698 ), #60717, .F. ) ;
#67900=EDGE_CURVE ( 'NONE', #49062, #36328, #50531, .T. ) ;
#67906=DIRECTION ( 'NONE',  ( 0.8225049752423776450, 0.5687579148473765889, -0.000000000000000000 ) ) ;
#67910=ADVANCED_FACE ( 'NONE', ( #39264 ), #67081, .F. ) ;
#67914=CARTESIAN_POINT ( 'NONE',  ( 2.874421927457452952, -143.3717286177755739, 5.500000000000000000 ) ) ;
#67926=CARTESIAN_POINT ( 'NONE',  ( -20.30386590532152979, -102.9045904027214959, 2.500000000000000000 ) ) ;
#67943=AXIS2_PLACEMENT_3D ( 'NONE', #29829, #36592, #70417 ) ;
#67963=VERTEX_POINT ( 'NONE', #50143 ) ;
#67970=ORIENTED_EDGE ( 'NONE', *, *, #68771, .F. ) ;
#68002=DIRECTION ( 'NONE',  ( -0.000000000000000000, -0.000000000000000000, -1.000000000000000000 ) ) ;
#68014=LINE ( 'NONE', #16507, #62855 ) ;
#68016=EDGE_CURVE ( 'NONE', #30226, #35224, #40004, .T. ) ;
#68040=EDGE_LOOP ( 'NONE', ( #55353, #68360, #52911, #1349 ) ) ;
#68047=ADVANCED_FACE ( 'NONE', ( #34349 ), #45660, .T. ) ;
#68048=VERTEX_POINT ( 'NONE', #29808 ) ;
#68057=DIRECTION ( 'NONE',  ( -1.000000000000000000, 0.000000000000000000, 0.000000000000000000 ) ) ;
#68058=EDGE_CURVE ( 'NONE', #8769, #37081, #71544, .T. ) ;
#68097=DIRECTION ( 'NONE',  ( -0.1045284632676570929, 0.9945218953682730678, 0.000000000000000000 ) ) ;
#68142=ORIENTED_EDGE ( 'NONE', *, *, #65801, .T. ) ;
#68146=FACE_OUTER_BOUND ( 'NONE', #70077, .T. ) ;
#68181=CARTESIAN_POINT ( 'NONE',  ( 16.84844760790522855, -103.5491698323862124, 5.500000000000000000 ) ) ;
#68206=DIRECTION ( 'NONE',  ( 0.000000000000000000, -0.000000000000000000, 1.000000000000000000 ) ) ;
#68208=VECTOR ( 'NONE', #36719, 1000.000000000000000 ) ;
#68212=VECTOR ( 'NONE', #61570, 1000.000000000000000 ) ;
#68239=ORIENTED_EDGE ( 'NONE', *, *, #73262, .F. ) ;
#68241=EDGE_CURVE ( 'NONE', #42731, #43669, #74017, .T. ) ;
#68255=DIRECTION ( 'NONE',  ( -0.000000000000000000, -0.000000000000000000, 1.000000000000000000 ) ) ;
#68284=VERTEX_POINT ( 'NONE', #38707 ) ;
#68289=DIRECTION ( 'NONE',  ( 0.000000000000000000, 0.000000000000000000, 1.000000000000000000 ) ) ;
#68320=LINE ( 'NONE', #22830, #4282 ) ;
#68323=EDGE_CURVE ( 'NONE', #30043, #52162, #16143, .T. ) ;
#68329=EDGE_CURVE ( 'NONE', #3158, #65921, #16893, .T. ) ;
#68334=PLANE ( 'NONE',  #29248 ) ;
#68350=ORIENTED_EDGE ( 'NONE', *, *, #44973, .F. ) ;
#68359=DIRECTION ( 'NONE',  ( -0.000000000000000000, -0.000000000000000000, -1.000000000000000000 ) ) ;
#68360=ORIENTED_EDGE ( 'NONE', *, *, #40158, .T. ) ;
#68413=CARTESIAN_POINT ( 'NONE',  ( 2.874421927457452952, -143.3717286177755739, -5.500000000000000000 ) ) ;
#68437=ORIENTED_EDGE ( 'NONE', *, *, #55233, .T. ) ;
#68444=LINE ( 'NONE', #57163, #4679 ) ;
#68458=VECTOR ( 'NONE', #54503, 1000.000000000000114 ) ;
#68560=CARTESIAN_POINT ( 'NONE',  ( -18.24502636017238899, -100.7225776329765665, 5.500000000000000000 ) ) ;
#68589=CARTESIAN_POINT ( 'NONE',  ( 25.81725066941077529, -113.8380548628854854, -5.500000000000000000 ) ) ;
#68652=PLANE ( 'NONE',  #24234 ) ;
#68657=PLANE ( 'NONE',  #34819 ) ;
#68682=DIRECTION ( 'NONE',  ( 0.9918136447140100120, -0.1276937514489704939, 0.000000000000000000 ) ) ;
#68691=VECTOR ( 'NONE', #47478, 1000.000000000000000 ) ;
#68771=EDGE_CURVE ( 'NONE', #40323, #52067, #29492, .T. ) ;
#68776=CARTESIAN_POINT ( 'NONE',  ( -0.8815729230226008184, -93.47222532549339746, 5.500000000000000000 ) ) ;
#68787=CARTESIAN_POINT ( 'NONE',  ( -0.9515373497862389396, -96.47140937769621871, -5.500000000000000000 ) ) ;
#68795=VERTEX_POINT ( 'NONE', #42288 ) ;
#68797=CARTESIAN_POINT ( 'NONE',  ( 2.874421927457452952, -143.3717286177755739, 5.500000000000000000 ) ) ;
#68804=DIRECTION ( 'NONE',  ( -0.7585478161175716050, -0.6516173805718067369, 0.000000000000000000 ) ) ;
#68869=DIRECTION ( 'NONE',  ( -0.8090169943749426773, -0.5877852522924797984, 0.000000000000000000 ) ) ;
#68902=VERTEX_POINT ( 'NONE', #34438 ) ;
#68911=ADVANCED_FACE ( 'NONE', ( #33703 ), #22054, .F. ) ;
#68933=VERTEX_POINT ( 'NONE', #53222 ) ;
#68935=ORIENTED_EDGE ( 'NONE', *, *, #3870, .T. ) ;
#68949=VECTOR ( 'NONE', #59605, 1000.000000000000227 ) ;
#68957=EDGE_CURVE ( 'NONE', #69250, #14710, #64140, .T. ) ;
#68964=PLANE ( 'NONE',  #61059 ) ;
#69025=VERTEX_POINT ( 'NONE', #41561 ) ;
#69065=LINE ( 'NONE', #1785, #25829 ) ;
#69077=ORIENTED_EDGE ( 'NONE', *, *, #2107, .F. ) ;
#69082=EDGE_CURVE ( 'NONE', #32596, #38564, #37424, .T. ) ;
#69091=LINE ( 'NONE', #28861, #3549 ) ;
#69109=VECTOR ( 'NONE', #35651, 999.9999999999998863 ) ;
#69129=EDGE_CURVE ( 'NONE', #1781, #48167, #44158, .T. ) ;
#69148=LINE ( 'NONE', #16156, #13123 ) ;
#69150=CARTESIAN_POINT ( 'NONE',  ( 5.822613034544236399, -142.8165987265839760, 5.500000000000000000 ) ) ;
#69170=DIRECTION ( 'NONE',  ( -0.000000000000000000, -0.000000000000000000, -1.000000000000000000 ) ) ;
#69193=ADVANCED_FACE ( 'NONE', ( #31383 ), #48684, .F. ) ;
#69227=DIRECTION ( 'NONE',  ( -0.000000000000000000, -0.000000000000000000, -1.000000000000000000 ) ) ;
#69233=PLANE ( 'NONE',  #39455 ) ;
#69250=VERTEX_POINT ( 'NONE', #68589 ) ;
#69255=VECTOR ( 'NONE', #40803, 1000.000000000000227 ) ;
#69310=VECTOR ( 'NONE', #49304, 1000.000000000000000 ) ;
#69344=LINE ( 'NONE', #58815, #3298 ) ;
#69381=ORIENTED_EDGE ( 'NONE', *, *, #54846, .T. ) ;
#69395=PLANE ( 'NONE',  #43347 ) ;
#69409=AXIS2_PLACEMENT_3D ( 'NONE', #5355, #33148, #38804 ) ;
#69420=VECTOR ( 'NONE', #55123, 1000.000000000000000 ) ;
#69445=ORIENTED_EDGE ( 'NONE', *, *, #39683, .T. ) ;
#69448=ADVANCED_FACE ( 'NONE', ( #58777 ), #46384, .F. ) ;
#69502=EDGE_CURVE ( 'NONE', #30226, #17504, #52011, .T. ) ;
#69511=EDGE_CURVE ( 'NONE', #37081, #8769, #11655, .T. ) ;
#69521=CARTESIAN_POINT ( 'NONE',  ( -21.33958957442910886, -129.9559990355020034, -2.500000000000000000 ) ) ;
#69538=CARTESIAN_POINT ( 'NONE',  ( 18.80329974962065265, -105.8248132807389084, 5.500000000000000000 ) ) ;
#69550=ORIENTED_EDGE ( 'NONE', *, *, #40648, .T. ) ;
#69562=DIRECTION ( 'NONE',  ( -0.3311129884571281101, -0.9435911131814402886, 0.000000000000000000 ) ) ;
#69577=DIRECTION ( 'NONE',  ( 0.4279312458753000703, 0.9038112904824842087, -0.000000000000000000 ) ) ;
#69584=VECTOR ( 'NONE', #38684, 1000.000000000000114 ) ;
#69600=FACE_OUTER_BOUND ( 'NONE', #36638, .T. ) ;
#69609=AXIS2_PLACEMENT_3D ( 'NONE', #13013, #43093, #61398 ) ;
#69613=AXIS2_PLACEMENT_3D ( 'NONE', #16303, #5044, #26832 ) ;
#69620=EDGE_CURVE ( 'NONE', #6205, #3158, #48951, .T. ) ;
#69623=ORIENTED_EDGE ( 'NONE', *, *, #20173, .T. ) ;
#69645=DIRECTION ( 'NONE',  ( 0.6691306063588671194, -0.7431448254773862505, 0.000000000000000000 ) ) ;
#69665=VERTEX_POINT ( 'NONE', #25304 ) ;
#69670=DIRECTION ( 'NONE',  ( -0.9227826878668540234, -0.3853207896976547642, 0.000000000000000000 ) ) ;
#69712=ORIENTED_EDGE ( 'NONE', *, *, #3529, .T. ) ;
#69788=PLANE ( 'NONE',  #64263 ) ;
#69793=CARTESIAN_POINT ( 'NONE',  ( 22.94323693612312809, -114.6983135802921083, 5.500000000000000000 ) ) ;
#69807=CARTESIAN_POINT ( 'NONE',  ( -1.029419772574582836, -121.0910063848724718, 2.500000000000000000 ) ) ;
#69827=ORIENTED_EDGE ( 'NONE', *, *, #6967, .T. ) ;
#69859=PLANE ( 'NONE',  #58972 ) ;
#69874=ORIENTED_EDGE ( 'NONE', *, *, #47381, .T. ) ;
#69877=ORIENTED_EDGE ( 'NONE', *, *, #46316, .F. ) ;
#69893=CARTESIAN_POINT ( 'NONE',  ( 0.000000000000000000, -120.0000000000000000, 5.500000000000000000 ) ) ;
#69900=ORIENTED_EDGE ( 'NONE', *, *, #30615, .F. ) ;
#69901=ORIENTED_EDGE ( 'NONE', *, *, #65178, .F. ) ;
#69909=ORIENTED_EDGE ( 'NONE', *, *, #57724, .F. ) ;
#69915=LINE ( 'NONE', #53014, #20490 ) ;
#69919=CARTESIAN_POINT ( 'NONE',  ( 6.377742925735834234, -145.7647898336708181, -5.500000000000000000 ) ) ;
#69930=LINE ( 'NONE', #29698, #35559 ) ;
#69944=EDGE_CURVE ( 'NONE', #10200, #45901, #63601, .T. ) ;
#69963=ORIENTED_EDGE ( 'NONE', *, *, #7067, .F. ) ;
#69976=FACE_OUTER_BOUND ( 'NONE', #39059, .T. ) ;
#69978=ORIENTED_EDGE ( 'NONE', *, *, #68016, .F. ) ;
#69983=ORIENTED_EDGE ( 'NONE', *, *, #58220, .T. ) ;
#69992=AXIS2_PLACEMENT_3D ( 'NONE', #29254, #28518, #11973 ) ;
#70006=ORIENTED_EDGE ( 'NONE', *, *, #19196, .T. ) ;
#70009=CARTESIAN_POINT ( 'NONE',  ( 0.000000000000000000, -120.0000000000000000, -2.500000000000000000 ) ) ;
#70014=CARTESIAN_POINT ( 'NONE',  ( 23.11608002360578240, -124.4885236261218182, 5.500000000000000000 ) ) ;
#70018=EDGE_LOOP ( 'NONE', ( #5232, #64269, #33358, #52628 ) ) ;
#70060=VERTEX_POINT ( 'NONE', #44643 ) ;
#70063=ORIENTED_EDGE ( 'NONE', *, *, #46316, .T. ) ;
#70072=LINE ( 'NONE', #18575, #67182 ) ;
#70077=EDGE_LOOP ( 'NONE', ( #45140, #54927, #22585, #21724 ) ) ;
#70078=CARTESIAN_POINT ( 'NONE',  ( 22.94323693612312809, -114.6983135802921083, 5.500000000000000000 ) ) ;
#70088=ADVANCED_FACE ( 'NONE', ( #38623 ), #30830, .T. ) ;
#70102=CARTESIAN_POINT ( 'NONE',  ( -1.233757462863590115, -120.8531368722710795, 2.500000000000000000 ) ) ;
#70106=VECTOR ( 'NONE', #43624, 1000.000000000000000 ) ;
#70119=EDGE_CURVE ( 'NONE', #12142, #34299, #32594, .T. ) ;
#70126=DIRECTION ( 'NONE',  ( 0.7585478161175723821, 0.6516173805718057377, 0.000000000000000000 ) ) ;
#70130=VECTOR ( 'NONE', #72780, 1000.000000000000114 ) ;
#70138=AXIS2_PLACEMENT_3D ( 'NONE', #69893, #41696, #47706 ) ;
#70177=EDGE_CURVE ( 'NONE', #36328, #44183, #34834, .T. ) ;
#70180=CARTESIAN_POINT ( 'NONE',  ( 20.85212586905261745, -130.9402397935870965, -2.500000000000000000 ) ) ;
#70192=ADVANCED_FACE ( 'NONE', ( #5907 ), #58127, .T. ) ;
#70242=VERTEX_POINT ( 'NONE', #54259 ) ;
#70254=ORIENTED_EDGE ( 'NONE', *, *, #16722, .T. ) ;
#70267=ORIENTED_EDGE ( 'NONE', *, *, #36314, .F. ) ;
#70324=DIRECTION ( 'NONE',  ( 0.6516173805718078471, -0.7585478161175706058, 0.000000000000000000 ) ) ;
#70332=LINE ( 'NONE', #2712, #62310 ) ;
#70369=EDGE_LOOP ( 'NONE', ( #34899, #71988, #43595, #70755 ) ) ;
#70381=( GEOMETRIC_REPRESENTATION_CONTEXT ( 3 ) GLOBAL_UNCERTAINTY_ASSIGNED_CONTEXT ( ( #48137 ) ) GLOBAL_UNIT_ASSIGNED_CONTEXT ( ( #12455, #35028, #854 ) ) REPRESENTATION_CONTEXT ( 'NONE', 'WORKASPACE' ) );
#70394=DIRECTION ( 'NONE',  ( -0.000000000000000000, -0.000000000000000000, 1.000000000000000000 ) ) ;
#70407=ADVANCED_FACE ( 'NONE', ( #74120 ), #28625, .F. ) ;
#70417=DIRECTION ( 'NONE',  ( -0.9997280174009349762, 0.02332147558787671729, 0.000000000000000000 ) ) ;
#70458=CARTESIAN_POINT ( 'NONE',  ( 6.377742925735834234, -145.7647898336708181, 5.500000000000000000 ) ) ;
#70466=PLANE ( 'NONE',  #64986 ) ;
#70484=CARTESIAN_POINT ( 'NONE',  ( -4.653126046682595884, -146.1313684676804314, 5.500000000000000000 ) ) ;
#70487=CARTESIAN_POINT ( 'NONE',  ( 9.984461079971730157, -95.40710393340120277, 5.500000000000000000 ) ) ;
#70500=ORIENTED_EDGE ( 'NONE', *, *, #24111, .T. ) ;
#70524=VERTEX_POINT ( 'NONE', #47768 ) ;
#70560=EDGE_LOOP ( 'NONE', ( #1811, #1599, #73063, #36411 ) ) ;
#70567=CARTESIAN_POINT ( 'NONE',  ( 2.047646702416564324, -96.54137380445985173, -2.500000000000000000 ) ) ;
#70583=FACE_OUTER_BOUND ( 'NONE', #56777, .T. ) ;
#70603=ORIENTED_EDGE ( 'NONE', *, *, #62909, .F. ) ;
#70611=ORIENTED_EDGE ( 'NONE', *, *, #18307, .T. ) ;
#70622=CARTESIAN_POINT ( 'NONE',  ( 24.95699195200416654, -110.9640411295978595, 5.500000000000000000 ) ) ;
#70627=DIRECTION ( 'NONE',  ( 0.5687579148473752566, -0.8225049752423786442, 0.000000000000000000 ) ) ;
#70636=FACE_BOUND ( 'NONE', #70369, .T. ) ;
#70674=LINE ( 'NONE', #52663, #3445 ) ;
#70703=ADVANCED_FACE ( 'NONE', ( #14297 ), #2326, .F. ) ;
#70707=FACE_BOUND ( 'NONE', #22504, .T. ) ;
#70711=ORIENTED_EDGE ( 'NONE', *, *, #40648, .F. ) ;
#70717=ORIENTED_EDGE ( 'NONE', *, *, #2107, .T. ) ;
#70719=EDGE_LOOP ( 'NONE', ( #13708, #28189, #47738, #49733 ) ) ;
#70733=ORIENTED_EDGE ( 'NONE', *, *, #52375, .T. ) ;
#70746=DIRECTION ( 'NONE',  ( 0.3853207896976547087, -0.9227826878668540234, 0.000000000000000000 ) ) ;
#70755=ORIENTED_EDGE ( 'NONE', *, *, #59013, .F. ) ;
#70763=CARTESIAN_POINT ( 'NONE',  ( 2.047646702416564768, -96.54137380445985173, 5.500000000000000000 ) ) ;
#70795=ORIENTED_EDGE ( 'NONE', *, *, #16105, .F. ) ;
#70800=ORIENTED_EDGE ( 'NONE', *, *, #46700, .F. ) ;
#70823=VERTEX_POINT ( 'NONE', #10895 ) ;
#70840=CARTESIAN_POINT ( 'NONE',  ( -4.653126046682595884, -146.1313684676804314, 5.500000000000000000 ) ) ;
#70910=VECTOR ( 'NONE', #47559, 1000.000000000000000 ) ;
#70925=DIRECTION ( 'NONE',  ( -0.7950889364178796992, 0.6064928550163511956, 0.000000000000000000 ) ) ;
#70940=VERTEX_POINT ( 'NONE', #22927 ) ;
#70941=CARTESIAN_POINT ( 'NONE',  ( -14.87942725330654348, -141.9795960975983178, 5.500000000000000000 ) ) ;
#70949=CARTESIAN_POINT ( 'NONE',  ( 22.08297821871651934, -111.8242998470044540, 2.500000000000000000 ) ) ;
#70952=LINE ( 'NONE', #36011, #27763 ) ;
#70974=DIRECTION ( 'NONE',  ( 0.1276937514489679681, 0.9918136447140103451, 0.000000000000000000 ) ) ;
#70978=ORIENTED_EDGE ( 'NONE', *, *, #61713, .T. ) ;
#70992=FACE_OUTER_BOUND ( 'NONE', #19407, .T. ) ;
#71003=LINE ( 'NONE', #152, #16518 ) ;
#71012=FACE_BOUND ( 'NONE', #22742, .T. ) ;
#71014=VERTEX_POINT ( 'NONE', #34551 ) ;
#71020=AXIS2_PLACEMENT_3D ( 'NONE', #52864, #53975, #7370 ) ;
#71032=CARTESIAN_POINT ( 'NONE',  ( 3.429551818649054340, -146.3199197248623875, 5.500000000000000000 ) ) ;
#71038=CARTESIAN_POINT ( 'NONE',  ( -14.87942725330654348, -141.9795960975983178, 5.500000000000000000 ) ) ;
#71045=LINE ( 'NONE', #8271, #24229 ) ;
#71057=DIRECTION ( 'NONE',  ( -0.9781476007338042455, -0.2079116908177664758, 0.000000000000000000 ) ) ;
#71063=PLANE ( 'NONE',  #54537 ) ;
#71076=VERTEX_POINT ( 'NONE', #69150 ) ;
#71113=DIRECTION ( 'NONE',  ( -0.5200609990132993854, -0.8541291221503275466, 0.000000000000000000 ) ) ;
#71117=DIRECTION ( 'NONE',  ( 0.08130631524010117905, -0.9966891607226784355, 0.000000000000000000 ) ) ;
#71128=DIRECTION ( 'NONE',  ( -0.000000000000000000, -0.000000000000000000, -1.000000000000000000 ) ) ;
#71133=DIRECTION ( 'NONE',  ( -0.2867529058022035837, 0.9580045777625452175, 0.000000000000000000 ) ) ;
#71157=VERTEX_POINT ( 'NONE', #36394 ) ;
#71184=DIRECTION ( 'NONE',  ( -0.2867529058022021404, 0.9580045777625456616, 0.000000000000000000 ) ) ;
#71204=FACE_OUTER_BOUND ( 'NONE', #18675, .T. ) ;
#71209=CARTESIAN_POINT ( 'NONE',  ( 26.47460221209471598, -121.8961639463267090, -5.500000000000000000 ) ) ;
#71218=AXIS2_PLACEMENT_3D ( 'NONE', #59457, #58711, #18481 ) ;
#71228=CARTESIAN_POINT ( 'NONE',  ( -0.1219594728601508804, -118.5049662589159567, 2.500000000000000000 ) ) ;
#71232=DIRECTION ( 'NONE',  ( 0.000000000000000000, 0.000000000000000000, 1.000000000000000000 ) ) ;
#71239=DIRECTION ( 'NONE',  ( 0.9435911131814395114, -0.3311129884571304971, 0.000000000000000000 ) ) ;
#71270=AXIS2_PLACEMENT_3D ( 'NONE', #66810, #60440, #37507 ) ;
#71308=ORIENTED_EDGE ( 'NONE', *, *, #60061, .T. ) ;
#71325=CIRCLE ( 'NONE', #54541, 30.50000000000000000 ) ;
#71331=ORIENTED_EDGE ( 'NONE', *, *, #67109, .T. ) ;
#71361=PLANE ( 'NONE',  #12559 ) ;
#71375=ADVANCED_FACE ( 'NONE', ( #28082 ), #67199, .T. ) ;
#71397=ORIENTED_EDGE ( 'NONE', *, *, #22772, .F. ) ;
#71493=LINE ( 'NONE', #65147, #10827 ) ;
#71509=LINE ( 'NONE', #37328, #17746 ) ;
#71539=CARTESIAN_POINT ( 'NONE',  ( 14.59956846177685996, -138.4757300459248484, -2.500000000000000000 ) ) ;
#71544=CIRCLE ( 'NONE', #43933, 35.50000000000000711 ) ;
#71546=ORIENTED_EDGE ( 'NONE', *, *, #56126, .F. ) ;
#71554=VERTEX_POINT ( 'NONE', #23712 ) ;
#71557=LINE ( 'NONE', #3176, #63283 ) ;
#71586=ORIENTED_EDGE ( 'NONE', *, *, #44482, .T. ) ;
#71617=ORIENTED_EDGE ( 'NONE', *, *, #73262, .T. ) ;
#71638=DIRECTION ( 'NONE',  ( 0.7273375899149802093, -0.6862798483830544471, 0.000000000000000000 ) ) ;
#71667=DIRECTION ( 'NONE',  ( -0.6862798483830544471, -0.7273375899149802093, 0.000000000000000000 ) ) ;
#71684=ADVANCED_FACE ( 'NONE', ( #4316 ), #38507, .T. ) ;
#71696=CARTESIAN_POINT ( 'NONE',  ( -24.50849501662245800, -109.8101191361138831, 5.500000000000000000 ) ) ;
#71708=CARTESIAN_POINT ( 'NONE',  ( -19.90058851926621131, -132.5883508287165853, -5.500000000000000000 ) ) ;
#71724=VERTEX_POINT ( 'NONE', #71038 ) ;
#71736=CARTESIAN_POINT ( 'NONE',  ( 26.09152095774781799, -124.8716048804687375, -5.500000000000000000 ) ) ;
#71747=FACE_OUTER_BOUND ( 'NONE', #776, .T. ) ;
#71756=ORIENTED_EDGE ( 'NONE', *, *, #303, .T. ) ;
#71786=LINE ( 'NONE', #26672, #70106 ) ;
#71789=CARTESIAN_POINT ( 'NONE',  ( -23.30023580412278505, -123.4057321492263384, 2.500000000000000000 ) ) ;
#71805=CARTESIAN_POINT ( 'NONE',  ( 12.69589495141918611, -96.69089767102708777, 5.500000000000000000 ) ) ;
#71813=EDGE_CURVE ( 'NONE', #11307, #24488, #31557, .T. ) ;
#71843=DIRECTION ( 'NONE',  ( -0.08130631524009862554, 0.9966891607226787686, 0.000000000000000000 ) ) ;
#71867=ADVANCED_FACE ( 'NONE', ( #54471 ), #8236, .F. ) ;
#71895=CARTESIAN_POINT ( 'NONE',  ( 16.30584220631899228, -140.9432449716519784, 5.500000000000000000 ) ) ;
#71904=CARTESIAN_POINT ( 'NONE',  ( 19.29194287201271862, -133.5026271600380880, -5.500000000000000000 ) ) ;
#71932=AXIS2_PLACEMENT_3D ( 'NONE', #61293, #55640, #61659 ) ;
#71959=ORIENTED_EDGE ( 'NONE', *, *, #66619, .F. ) ;
#71967=EDGE_CURVE ( 'NONE', #18041, #37728, #49566, .T. ) ;
#71986=FACE_OUTER_BOUND ( 'NONE', #57619, .T. ) ;
#71988=ORIENTED_EDGE ( 'NONE', *, *, #70119, .F. ) ;
#71993=VECTOR ( 'NONE', #67511, 1000.000000000000114 ) ;
#72000=EDGE_LOOP ( 'NONE', ( #50283, #40311, #24212, #52504 ) ) ;
#72008=CARTESIAN_POINT ( 'NONE',  ( -7.670864526094547386, -97.73662565058241114, -2.500000000000000000 ) ) ;
#72023=EDGE_CURVE ( 'NONE', #53084, #45726, #65402, .T. ) ;
#72028=ORIENTED_EDGE ( 'NONE', *, *, #38968, .T. ) ;
#72033=VERTEX_POINT ( 'NONE', #33769 ) ;
#72041=VECTOR ( 'NONE', #46095, 999.9999999999998863 ) ;
#72074=LINE ( 'NONE', #71696, #10579 ) ;
#72090=AXIS2_PLACEMENT_3D ( 'NONE', #62072, #72218, #20722 ) ;
#72091=CARTESIAN_POINT ( 'NONE',  ( -6.880223345695647197, -142.5202692415819854, -5.500000000000000000 ) ) ;
#72099=LINE ( 'NONE', #37902, #64174 ) ;
#72109=CARTESIAN_POINT ( 'NONE',  ( 22.51310757741980240, -113.2613067136482101, -2.500000000000000000 ) ) ;
#72123=ORIENTED_EDGE ( 'NONE', *, *, #62951, .T. ) ;
#72169=LINE ( 'NONE', #3778, #50590 ) ;
#72171=LINE ( 'NONE', #43992, #8862 ) ;
#72177=AXIS2_PLACEMENT_3D ( 'NONE', #51997, #549, #69670 ) ;
#72187=ORIENTED_EDGE ( 'NONE', *, *, #36343, .F. ) ;
#72189=ORIENTED_EDGE ( 'NONE', *, *, #5276, .F. ) ;
#72218=DIRECTION ( 'NONE',  ( 0.000000000000000000, 0.000000000000000000, -1.000000000000000000 ) ) ;
#72248=CARTESIAN_POINT ( 'NONE',  ( 5.822613034544236399, -142.8165987265839760, 5.500000000000000000 ) ) ;
#72258=DIRECTION ( 'NONE',  ( -0.000000000000000000, 0.000000000000000000, -1.000000000000000000 ) ) ;
#72266=DIRECTION ( 'NONE',  ( -0.9966891607226786576, -0.08130631524009861166, 0.000000000000000000 ) ) ;
#72283=VECTOR ( 'NONE', #42483, 1000.000000000000114 ) ;
#72307=VECTOR ( 'NONE', #8082, 1000.000000000000000 ) ;
#72316=DIRECTION ( 'NONE',  ( -0.02332147558787823344, -0.9997280174009349762, 0.000000000000000000 ) ) ;
#72336=EDGE_LOOP ( 'NONE', ( #36433, #11143, #32451, #46576 ) ) ;
#72339=ADVANCED_FACE ( 'NONE', ( #55129 ), #42378, .F. ) ;
#72343=CARTESIAN_POINT ( 'NONE',  ( 19.12409105625795291, -101.5943176906707919, 5.500000000000000000 ) ) ;
#72351=DIRECTION ( 'NONE',  ( 0.9966891607226785466, 0.08130631524009969413, -0.000000000000000000 ) ) ;
#72388=ORIENTED_EDGE ( 'NONE', *, *, #61397, .F. ) ;
#72390=VECTOR ( 'NONE', #54446, 1000.000000000000000 ) ;
#72403=ORIENTED_EDGE ( 'NONE', *, *, #66112, .F. ) ;
#72411=DIRECTION ( 'NONE',  ( -0.000000000000000000, -0.000000000000000000, -1.000000000000000000 ) ) ;
#72427=CARTESIAN_POINT ( 'NONE',  ( 12.69589495141918611, -96.69089767102708777, -2.500000000000000444 ) ) ;
#72441=PRODUCT_DEFINITION_CONTEXT ( 'detailed design', #56092, 'design' ) ;
#72455=ADVANCED_FACE ( 'NONE', ( #15276 ), #66428, .F. ) ;
#72479=CARTESIAN_POINT ( 'NONE',  ( 0.6180191030787338669, -93.50720753887522108, 2.500000000000000000 ) ) ;
#72485=EDGE_CURVE ( 'NONE', #21360, #70060, #61156, .T. ) ;
#72486=CARTESIAN_POINT ( 'NONE',  ( 23.11608002360578240, -124.4885236261218182, 5.500000000000000000 ) ) ;
#72494=CARTESIAN_POINT ( 'NONE',  ( -21.67772167707813935, -110.8034581014852762, 5.500000000000000000 ) ) ;
#72510=DIRECTION ( 'NONE',  ( 0.2867529058022035837, -0.9580045777625452175, 0.000000000000000000 ) ) ;
#72520=DIRECTION ( 'NONE',  ( 0.8225049752423776450, 0.5687579148473764779, 0.000000000000000000 ) ) ;
#72542=EDGE_LOOP ( 'NONE', ( #52715, #23802, #27083, #17542 ) ) ;
#72557=ORIENTED_EDGE ( 'NONE', *, *, #54555, .F. ) ;
#72574=ORIENTED_EDGE ( 'NONE', *, *, #64209, .F. ) ;
#72580=ORIENTED_EDGE ( 'NONE', *, *, #33635, .F. ) ;
#72619=ORIENTED_EDGE ( 'NONE', *, *, #13473, .F. ) ;
#72639=CARTESIAN_POINT ( 'NONE',  ( 1.029419772574596825, -118.9089936151275140, 2.500000000000000000 ) ) ;
#72640=ORIENTED_EDGE ( 'NONE', *, *, #49841, .F. ) ;
#72641=DIRECTION ( 'NONE',  ( 0.000000000000000000, -0.000000000000000000, 1.000000000000000000 ) ) ;
#72698=FACE_BOUND ( 'NONE', #3908, .T. ) ;
#72702=CARTESIAN_POINT ( 'NONE',  ( 12.69589495141918611, -96.69089767102708777, 5.500000000000000000 ) ) ;
#72724=EDGE_CURVE ( 'NONE', #24993, #22209, #54222, .T. ) ;
#72725=ORIENTED_EDGE ( 'NONE', *, *, #66380, .F. ) ;
#72735=ORIENTED_EDGE ( 'NONE', *, *, #22772, .T. ) ;
#72744=EDGE_LOOP ( 'NONE', ( #65867, #25410, #7100, #6480 ) ) ;
#72745=ADVANCED_FACE ( 'NONE', ( #19985 ), #59862, .F. ) ;
#72749=DIRECTION ( 'NONE',  ( 0.7950889364178788110, -0.6064928550163524168, 0.000000000000000000 ) ) ;
#72770=CARTESIAN_POINT ( 'NONE',  ( 12.69589495141918611, -96.69089767102708777, -5.500000000000000000 ) ) ;
#72772=ORIENTED_EDGE ( 'NONE', *, *, #4513, .T. ) ;
#72780=DIRECTION ( 'NONE',  ( 0.5687579148473743684, -0.8225049752423791993, 0.000000000000000000 ) ) ;
#72793=CARTESIAN_POINT ( 'NONE',  ( 23.49916127795269460, -121.5130826919798039, 5.500000000000000000 ) ) ;
#72842=ORIENTED_EDGE ( 'NONE', *, *, #49659, .F. ) ;
#72843=DIRECTION ( 'NONE',  ( -0.000000000000000000, -0.000000000000000000, -1.000000000000000000 ) ) ;
#72846=ORIENTED_EDGE ( 'NONE', *, *, #58382, .F. ) ;
#72924=EDGE_LOOP ( 'NONE', ( #13381, #20868, #36795, #59764 ) ) ;
#72966=ORIENTED_EDGE ( 'NONE', *, *, #9253, .F. ) ;
#72975=ADVANCED_FACE ( 'NONE', ( #60713 ), #9192, .F. ) ;
#73005=FACE_OUTER_BOUND ( 'NONE', #25624, .T. ) ;
#73025=DIRECTION ( 'NONE',  ( 0.000000000000000000, -0.000000000000000000, 1.000000000000000000 ) ) ;
#73038=VECTOR ( 'NONE', #51925, 1000.000000000000114 ) ;
#73049=ORIENTED_EDGE ( 'NONE', *, *, #20653, .T. ) ;
#73051=DIRECTION ( 'NONE',  ( 0.000000000000000000, 0.000000000000000000, 1.000000000000000000 ) ) ;
#73063=ORIENTED_EDGE ( 'NONE', *, *, #56479, .F. ) ;
#73075=ORIENTED_EDGE ( 'NONE', *, *, #47626, .T. ) ;
#73087=AXIS2_PLACEMENT_3D ( 'NONE', #3180, #71184, #25348 ) ;
#73091=VECTOR ( 'NONE', #58218, 1000.000000000000000 ) ;
#73112=AXIS2_PLACEMENT_3D ( 'NONE', #29291, #18027, #24048 ) ;
#73122=FACE_OUTER_BOUND ( 'NONE', #72000, .T. ) ;
#73146=LINE ( 'NONE', #70458, #43396 ) ;
#73148=CARTESIAN_POINT ( 'NONE',  ( -14.25258209288423750, -138.6845900058201551, -2.500000000000000000 ) ) ;
#73165=DIRECTION ( 'NONE',  ( -0.5000000000000039968, 0.8660254037844363761, 0.000000000000000000 ) ) ;
#73188=EDGE_CURVE ( 'NONE', #46917, #17376, #40362, .T. ) ;
#73248=VERTEX_POINT ( 'NONE', #17790 ) ;
#73256=CARTESIAN_POINT ( 'NONE',  ( -25.50183398199384754, -112.6408924756582053, 5.500000000000000000 ) ) ;
#73257=CARTESIAN_POINT ( 'NONE',  ( -30.50000000000000000, -120.0000000000000000, 2.500000000000000000 ) ) ;
#73259=DIRECTION ( 'NONE',  ( 0.9918136447140104561, -0.1276937514489679681, 0.000000000000000000 ) ) ;
#73262=EDGE_CURVE ( 'NONE', #56886, #33390, #923, .T. ) ;
#73264=AXIS2_PLACEMENT_3D ( 'NONE', #37930, #26637, #48827 ) ;
#73279=AXIS2_PLACEMENT_3D ( 'NONE', #67332, #71843, #55681 ) ;
#73280=LINE ( 'NONE', #61647, #47881 ) ;
#73290=ORIENTED_EDGE ( 'NONE', *, *, #15029, .T. ) ;
#73298=EDGE_CURVE ( 'NONE', #21360, #19317, #43243, .T. ) ;
#73327=FACE_BOUND ( 'NONE', #61824, .T. ) ;
#73378=AXIS2_PLACEMENT_3D ( 'NONE', #32128, #44171, #49791 ) ;
#73393=ORIENTED_EDGE ( 'NONE', *, *, #58664, .F. ) ;
#73426=VECTOR ( 'NONE', #36720, 1000.000000000000000 ) ;
#73476=EDGE_CURVE ( 'NONE', #45237, #26049, #20002, .T. ) ;
#73483=EDGE_CURVE ( 'NONE', #16194, #52621, #17253, .T. ) ;
#73502=PLANE ( 'NONE',  #55009 ) ;
#73528=FACE_OUTER_BOUND ( 'NONE', #36798, .T. ) ;
#73535=CARTESIAN_POINT ( 'NONE',  ( -26.29030328629082902, -123.6496510949466341, -2.500000000000000000 ) ) ;
#73546=DIRECTION ( 'NONE',  ( 0.9038112904824842087, -0.4279312458753000703, 0.000000000000000000 ) ) ;
#73564=DIRECTION ( 'NONE',  ( -0.000000000000000000, -0.000000000000000000, 1.000000000000000000 ) ) ;
#73589=CARTESIAN_POINT ( 'NONE',  ( 48.80839716909466830, -10.37454508288725208, 5.500000000000000000 ) ) ;
#73620=VECTOR ( 'NONE', #18717, 1000.000000000000000 ) ;
#73636=CARTESIAN_POINT ( 'NONE',  ( 5.822613034544236399, -142.8165987265839760, 5.500000000000000000 ) ) ;
#73650=EDGE_CURVE ( 'NONE', #11562, #22041, #57114, .T. ) ;
#73654=FACE_OUTER_BOUND ( 'NONE', #60116, .T. ) ;
#73658=DIRECTION ( 'NONE',  ( -0.6862798483830534479, -0.7273375899149810975, 0.000000000000000000 ) ) ;
#73688=DIRECTION ( 'NONE',  ( -0.5200609990132993854, -0.8541291221503275466, 0.000000000000000000 ) ) ;
#73732=EDGE_CURVE ( 'NONE', #32752, #34951, #13808, .T. ) ;
#73742=DIRECTION ( 'NONE',  ( 0.2867529058022011967, -0.9580045777625459946, 0.000000000000000000 ) ) ;
#73744=DIRECTION ( 'NONE',  ( -0.000000000000000000, -0.000000000000000000, -1.000000000000000000 ) ) ;
#73766=EDGE_CURVE ( 'NONE', #8717, #57544, #19822, .T. ) ;
#73777=FACE_OUTER_BOUND ( 'NONE', #70018, .T. ) ;
#73780=VERTEX_POINT ( 'NONE', #72793 ) ;
#73797=ORIENTED_EDGE ( 'NONE', *, *, #39337, .T. ) ;
#73828=DIRECTION ( 'NONE',  ( 1.000000000000000000, 0.000000000000000000, 0.000000000000000000 ) ) ;
#73837=DIRECTION ( 'NONE',  ( 0.5687579148473744795, -0.8225049752423790883, 0.000000000000000000 ) ) ;
#73846=ORIENTED_EDGE ( 'NONE', *, *, #62993, .F. ) ;
#73850=AXIS2_PLACEMENT_3D ( 'NONE', #41223, #1043, #57782 ) ;
#73870=VECTOR ( 'NONE', #56157, 1000.000000000000114 ) ;
#73880=CARTESIAN_POINT ( 'NONE',  ( -6.112675177960399608, -145.7853679859090903, 2.500000000000000000 ) ) ;
#73904=EDGE_LOOP ( 'NONE', ( #24990, #1653, #69381, #48840 ) ) ;
#73909=CARTESIAN_POINT ( 'NONE',  ( 11.41210121379328335, -99.40233154247455616, 5.500000000000000000 ) ) ;
#73914=ORIENTED_EDGE ( 'NONE', *, *, #16716, .F. ) ;
#73933=DIRECTION ( 'NONE',  ( 0.9730327541852497042, -0.2306669878475622604, 0.000000000000000000 ) ) ;
#73942=DIRECTION ( 'NONE',  ( 0.9966891607226786576, 0.08130631524009862554, 0.000000000000000000 ) ) ;
#73954=VECTOR ( 'NONE', #2755, 1000.000000000000000 ) ;
#73958=EDGE_LOOP ( 'NONE', ( #42353, #51565, #6346, #6611 ) ) ;
#73965=AXIS2_PLACEMENT_3D ( 'NONE', #32117, #62192, #5067 ) ;
#74017=LINE ( 'NONE', #33805, #9203 ) ;
#74028=ADVANCED_FACE ( 'NONE', ( #5162 ), #11510, .F. ) ;
#74029=EDGE_CURVE ( 'NONE', #49489, #14738, #34947, .T. ) ;
#74039=ORIENTED_EDGE ( 'NONE', *, *, #38096, .T. ) ;
#74055=FACE_OUTER_BOUND ( 'NONE', #43269, .T. ) ;
#74081=VECTOR ( 'NONE', #30731, 1000.000000000000000 ) ;
#74108=EDGE_CURVE ( 'NONE', #38564, #973, #64883, .T. ) ;
#74119=CARTESIAN_POINT ( 'NONE',  ( 24.95699195200416654, -110.9640411295978595, 5.500000000000000000 ) ) ;
#74120=FACE_OUTER_BOUND ( 'NONE', #16086, .T. ) ;
#74137=EDGE_LOOP ( 'NONE', ( #2808, #3096, #5669, #21257 ) ) ;
#74138=PLANE ( 'NONE',  #27402 ) ;
#74154=ORIENTED_EDGE ( 'NONE', *, *, #42132, .T. ) ;
#74186=DIRECTION ( 'NONE',  ( 0.9918136447140100120, -0.1276937514489704939, 0.000000000000000000 ) ) ;
#74196=LINE ( 'NONE', #64043, #62227 ) ;
#74231=VECTOR ( 'NONE', #71133, 1000.000000000000114 ) ;
#74234=AXIS2_PLACEMENT_3D ( 'NONE', #4805, #37240, #42142 ) ;
#74245=ORIENTED_EDGE ( 'NONE', *, *, #50023, .F. ) ;
#74247=DIRECTION ( 'NONE',  ( 0.9580045777625456616, 0.2867529058022021404, 0.000000000000000000 ) ) ;
#74251=ADVANCED_FACE ( 'NONE', ( #648 ), #24647, .F. ) ;
#74259=ADVANCED_FACE ( 'NONE', ( #52106 ), #69395, .F. ) ;
#74272=DIRECTION ( 'NONE',  ( 0.9997280174009349762, -0.02332147558787671729, 0.000000000000000000 ) ) ;
#74285=CARTESIAN_POINT ( 'NONE',  ( -7.670864526094549163, -97.73662565058241114, 5.500000000000000000 ) ) ;
#74287=DIRECTION ( 'NONE',  ( -0.9918136447140104561, 0.1276937514489679681, 0.000000000000000000 ) ) ;
#74326=EDGE_LOOP ( 'NONE', ( #16025, #70795, #13148, #48551 ) ) ;
ENDSEC;
END-ISO-10303-21;
